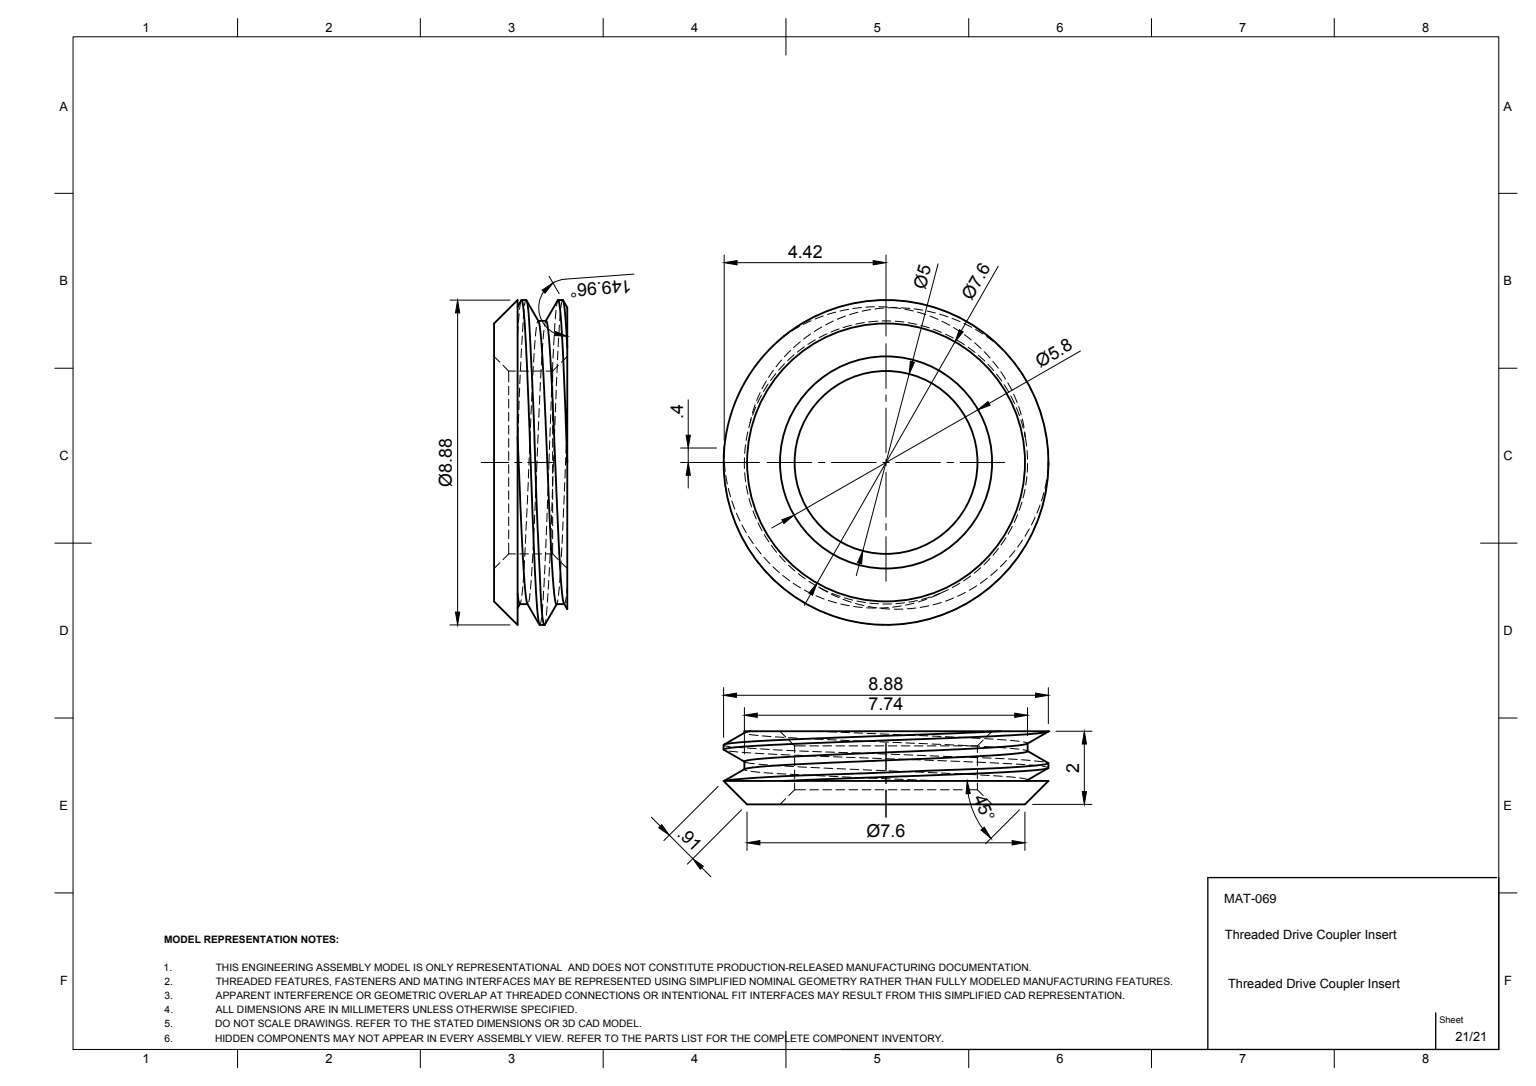
ISO-10303-21;
HEADER;
/* Generated by software containing ST-Developer
 * from STEP Tools, Inc. (www.steptools.com) 
 */

FILE_DESCRIPTION(
/* description */ ('CAx-IF Rec.Pracs.---Representation and Presentation of Product Manufa
cturing Information (PMI)---4.0---2014-10-13'),
/* implementation_level */ '2;1');

FILE_NAME(
/* name */ 'Threaded Drive Coupler Insert.step',
/* time_stamp */ '2026-10-24T15:08:39-07:00',
/* author */ (''),
/* organization */ (''),
/* preprocessor_version */ 'ST-DEVELOPER v20.2',
/* originating_system */ 'Autodesk Translation Framework v15.17.0.0',
/* authorisation */ '');

FILE_SCHEMA (('AP242_MANAGED_MODEL_BASED_3D_ENGINEERING_MIM_LF { 1 0 10303 442 2 1 4 }'));
ENDSEC;

DATA;
#10=MECHANICAL_DESIGN_GEOMETRIC_PRESENTATION_REPRESENTATION('',(#839),#50081);
#139=B_SPLINE_SURFACE_WITH_KNOTS('',3,3,((#49898,#49899,#49900,#49901,#49902,
#49903,#49904,#49905,#49906,#49907,#49908,#49909,#49910,#49911),(#49912,
#49913,#49914,#49915,#49916,#49917,#49918,#49919,#49920,#49921,#49922,#49923,
#49924,#49925),(#49926,#49927,#49928,#49929,#49930,#49931,#49932,#49933,
#49934,#49935,#49936,#49937,#49938,#49939),(#49940,#49941,#49942,#49943,
#49944,#49945,#49946,#49947,#49948,#49949,#49950,#49951,#49952,#49953)),
 .UNSPECIFIED.,.F.,.F.,.F.,(4,4),(4,1,1,1,1,1,1,1,1,1,1,4),(-0.000475468026429485,
0.0667497669206857),(7.06827384690996,8.03224682715675,8.99591018373647,
9.95957354031619,10.9232368968959,11.8869002534756,12.8505636100553,13.8142269666351,
14.7778903232148,15.7415536797945,16.7052170363742,17.6690343848084),
 .UNSPECIFIED.);
#140=B_SPLINE_SURFACE_WITH_KNOTS('',3,3,((#49960,#49961,#49962,#49963,#49964,
#49965,#49966,#49967,#49968,#49969,#49970,#49971,#49972,#49973),(#49974,
#49975,#49976,#49977,#49978,#49979,#49980,#49981,#49982,#49983,#49984,#49985,
#49986,#49987),(#49988,#49989,#49990,#49991,#49992,#49993,#49994,#49995,
#49996,#49997,#49998,#49999,#50000,#50001),(#50002,#50003,#50004,#50005,
#50006,#50007,#50008,#50009,#50010,#50011,#50012,#50013,#50014,#50015)),
 .UNSPECIFIED.,.F.,.F.,.F.,(4,4),(4,1,1,1,1,1,1,1,1,1,1,4),(-0.000976054051980672,
0.0662815922873265),(10.4983829434381,11.4623026957119,12.4259660522916,
13.3896294088713,14.353292765451,15.3169561220308,16.2806194786105,17.2442828351902,
18.2079461917699,19.1716095483496,20.1352729049293,21.0993547069101),
 .UNSPECIFIED.);
#588=B_SPLINE_CURVE_WITH_KNOTS('',3,(#49306,#49307,#49308,#49309,#49310,
#49311,#49312,#49313,#49314,#49315,#49316,#49317,#49318,#49319,#49320,#49321,
#49322,#49323,#49324,#49325,#49326,#49327,#49328,#49329,#49330),
 .UNSPECIFIED.,.F.,.F.,(4,3,3,3,3,3,3,3,4),(0.,0.160731090032336,0.25,0.407767129262868,
0.5,0.657767129262875,0.75,0.910731090032353,1.),.UNSPECIFIED.);
#589=B_SPLINE_CURVE_WITH_KNOTS('',3,(#49333,#49334,#49335,#49336,#49337,
#49338,#49339),.UNSPECIFIED.,.F.,.F.,(4,1,1,1,4),(0.,0.25,0.5,0.75,0.999999761822425),
 .UNSPECIFIED.);
#590=B_SPLINE_CURVE_WITH_KNOTS('',3,(#49345,#49346,#49347,#49348,#49349,
#49350,#49351,#49352,#49353,#49354,#49355,#49356,#49357,#49358,#49359,#49360,
#49361,#49362,#49363,#49364,#49365,#49366,#49367,#49368,#49369,#49370,#49371,
#49372,#49373,#49374,#49375,#49376,#49377,#49378,#49379,#49380,#49381,#49382,
#49383,#49384),.UNSPECIFIED.,.F.,.F.,(4,3,3,3,3,3,3,3,3,3,3,3,3,4),(0.235508041128149,
0.25,0.331910603091831,0.375,0.456895223609452,0.5,0.581895223609489,0.625,
0.706910603091898,0.75,0.831608731491742,0.875,0.958140783942944,0.999999441342508),
 .UNSPECIFIED.);
#591=B_SPLINE_CURVE_WITH_KNOTS('',3,(#49386,#49387,#49388,#49389),
 .UNSPECIFIED.,.F.,.F.,(4,4),(0.,0.987035809516257),.UNSPECIFIED.);
#592=B_SPLINE_CURVE_WITH_KNOTS('',3,(#49392,#49393,#49394,#49395,#49396,
#49397,#49398,#49399,#49400,#49401,#49402,#49403,#49404,#49405,#49406,#49407,
#49408,#49409,#49410,#49411,#49412,#49413,#49414,#49415),.UNSPECIFIED.,
 .F.,.F.,(4,2,2,2,2,2,2,2,2,2,2,4),(0.,0.100888900202487,0.125,0.22459286542628,
0.25,0.349878675008739,0.375,0.474842812735284,0.5,0.599842812735286,0.625,
0.715961029345133),.UNSPECIFIED.);
#593=B_SPLINE_CURVE_WITH_KNOTS('',3,(#49418,#49419,#49420,#49421,#49422,
#49423,#49424,#49425,#49426,#49427,#49428,#49429,#49430,#49431,#49432,#49433),
 .UNSPECIFIED.,.F.,.F.,(4,3,3,3,3,4),(0.715961029345133,0.75,0.849592865426306,
0.875,0.975888900203264,1.),.UNSPECIFIED.);
#594=B_SPLINE_CURVE_WITH_KNOTS('',3,(#49435,#49436,#49437,#49438,#49439,
#49440,#49441,#49442,#49443,#49444,#49445,#49446,#49447,#49448,#49449,#49450,
#49451,#49452,#49453,#49454,#49455,#49456,#49457,#49458,#49459),
 .UNSPECIFIED.,.F.,.F.,(4,3,3,3,3,3,3,3,4),(1.51276851349366E-6,0.156898311431348,
0.25,0.403657035544793,0.5,0.653657035544841,0.75,0.906896809192571,1.),
 .UNSPECIFIED.);
#595=B_SPLINE_CURVE_WITH_KNOTS('',3,(#49463,#49464,#49465,#49466,#49467,
#49468,#49469,#49470,#49471,#49472,#49473,#49474,#49475,#49476,#49477,#49478,
#49479,#49480,#49481),.UNSPECIFIED.,.F.,.F.,(4,3,3,3,3,3,4),(0.,0.25,0.491380882785342,
0.5,0.75,0.982966826876961,1.),.UNSPECIFIED.);
#596=B_SPLINE_CURVE_WITH_KNOTS('',3,(#49482,#49483,#49484,#49485,#49486,
#49487,#49488,#49489,#49490,#49491),.UNSPECIFIED.,.F.,.F.,(4,2,2,2,4),(0.,
0.0831407875458867,0.125,0.206497666001318,0.235508041094431),
 .UNSPECIFIED.);
#597=B_SPLINE_CURVE_WITH_KNOTS('',3,(#49494,#49495,#49496,#49497,#49498,
#49499,#49500,#49501,#49502,#49503,#49504,#49505,#49506,#49507,#49508,#49509,
#49510,#49511,#49512,#49513,#49514,#49515,#49516,#49517,#49518,#49519,#49520,
#49521,#49522,#49523,#49524,#49525,#49526,#49527,#49528,#49529,#49530,#49531,
#49532,#49533,#49534,#49535,#49536,#49537,#49538,#49539,#49540,#49541,#49542,
#49543,#49544,#49545,#49546,#49547,#49548,#49549,#49550,#49551,#49552,#49553,
#49554,#49555,#49556,#49557,#49558,#49559,#49560,#49561,#49562,#49563,#49564,
#49565,#49566,#49567,#49568,#49569,#49570,#49571,#49572,#49573,#49574,#49575,
#49576,#49577,#49578,#49579,#49580,#49581,#49582,#49583,#49584,#49585,#49586,
#49587,#49588,#49589),.UNSPECIFIED.,.F.,.F.,(4,2,2,2,2,2,2,2,2,2,2,2,2,
2,2,2,2,2,2,2,2,2,2,2,2,2,2,2,2,2,2,2,2,2,2,2,2,2,2,2,2,2,2,2,2,2,2,4),
(0.000203483817492821,0.0274848173325521,0.0563713830966491,0.167677917602274,
0.208184918082086,0.239301283250976,0.272826962459817,0.365270654699785,
0.43178988571008,0.47678039384355,0.587559073236576,0.632135152418474,0.664943612441571,
0.694797097900161,0.799548600392106,0.862971031190955,0.907614126172384,
0.988296557870209,1.06800029357004,1.09774395705088,1.13107244772413,1.22338481693792,
1.27276714107893,1.31911661255326,1.37385993664007,1.44604280082289,1.50302473070022,
1.53055325884595,1.56982870717352,1.63222593298961,1.71178156213431,1.75641486537916,
1.81980681943984,1.92449539617685,1.95434391906131,1.98714005868704,2.03169939876711,
2.14252612578957,2.18750485709249,2.25402546067906,2.3464077625176,2.37990009772018,
2.41102584148667,2.45156693199543,2.56907534347477,2.61465490234983,2.68897499185438,
2.74712781989908),.UNSPECIFIED.);
#598=B_SPLINE_CURVE_WITH_KNOTS('',3,(#49592,#49593,#49594,#49595,#49596,
#49597,#49598,#49599,#49600,#49601,#49602),.UNSPECIFIED.,.F.,.F.,(4,1,1,
1,1,1,1,1,4),(0.,0.125,0.25,0.375,0.5,0.625,0.75,0.875,0.999999067031556),
 .UNSPECIFIED.);
#599=B_SPLINE_CURVE_WITH_KNOTS('',3,(#49615,#49616,#49617,#49618,#49619,
#49620,#49621,#49622,#49623,#49624,#49625,#49626,#49627,#49628,#49629,#49630,
#49631,#49632,#49633,#49634,#49635,#49636,#49637,#49638,#49639,#49640,#49641,
#49642,#49643,#49644,#49645,#49646,#49647,#49648,#49649,#49650,#49651,#49652,
#49653,#49654,#49655,#49656,#49657,#49658,#49659,#49660,#49661,#49662,#49663,
#49664,#49665,#49666,#49667,#49668,#49669,#49670,#49671,#49672,#49673,#49674,
#49675,#49676,#49677,#49678,#49679,#49680,#49681,#49682,#49683,#49684,#49685,
#49686,#49687,#49688,#49689,#49690,#49691,#49692,#49693,#49694,#49695,#49696,
#49697,#49698,#49699,#49700,#49701,#49702,#49703,#49704,#49705),
 .UNSPECIFIED.,.F.,.F.,(4,3,3,3,3,3,3,3,3,3,3,3,3,3,3,3,3,3,3,3,3,3,3,3,
3,3,3,3,3,3,4),(0.,0.0549095480248197,0.0909168947914259,0.127664846372719,
0.147588217015191,0.152802982426264,0.157890055006788,0.195093310789768,
0.232935081254819,0.292943797457197,0.305066964469618,0.310416184503556,
0.349172960287603,0.387949178487593,0.446438776652271,0.460993647480443,
0.469743525078789,0.474867539044195,0.512454117005302,0.550939413816203,
0.624355350952517,0.633225532922949,0.64024307789027,0.680180338798595,
0.720316379107474,0.73809145220851,0.748199996374111,0.754956026360989,
0.795541316014259,0.835496820076563,0.862516963915765),.UNSPECIFIED.);
#600=B_SPLINE_CURVE_WITH_KNOTS('',3,(#49706,#49707,#49708,#49709,#49710,
#49711,#49712,#49713,#49714,#49715,#49716,#49717,#49718,#49719,#49720,#49721,
#49722,#49723,#49724,#49725,#49726,#49727,#49728,#49729,#49730,#49731,#49732,
#49733,#49734,#49735,#49736,#49737,#49738,#49739,#49740,#49741,#49742,#49743,
#49744,#49745,#49746,#49747,#49748,#49749,#49750,#49751,#49752,#49753,#49754,
#49755,#49756,#49757,#49758,#49759,#49760,#49761,#49762,#49763,#49764,#49765,
#49766,#49767,#49768,#49769,#49770,#49771,#49772),.UNSPECIFIED.,.F.,.F.,
(4,3,3,3,3,3,3,3,3,3,3,3,3,3,3,3,3,3,3,3,3,3,4),(0.,0.0399225644477167,
0.0623885722514162,0.164012510354697,0.170043304514999,0.174785078605868,
0.294020040644772,0.316832921701425,0.3295965682445,0.337876395007978,0.382194010439746,
0.420601788797671,0.476523089097994,0.50063461453704,0.506312621506711,
0.652610410209141,0.659762241707176,0.665735072710524,0.763244547674934,
0.769629684943624,0.806337248425914,0.842085556810208,0.865008878888598),
 .UNSPECIFIED.);
#601=B_SPLINE_CURVE_WITH_KNOTS('',3,(#49773,#49774,#49775,#49776,#49777,
#49778),.UNSPECIFIED.,.F.,.F.,(4,2,4),(3.98711970495987E-6,0.000952908437083531,
0.00170790873623591),.UNSPECIFIED.);
#602=B_SPLINE_CURVE_WITH_KNOTS('',3,(#49790,#49791,#49792,#49793,#49794,
#49795,#49796,#49797,#49798,#49799,#49800,#49801,#49802,#49803,#49804,#49805,
#49806,#49807,#49808,#49809,#49810,#49811,#49812,#49813,#49814,#49815,#49816,
#49817,#49818,#49819,#49820,#49821,#49822,#49823,#49824,#49825,#49826,#49827,
#49828,#49829,#49830,#49831,#49832,#49833,#49834,#49835,#49836,#49837,#49838,
#49839,#49840,#49841,#49842,#49843,#49844),.UNSPECIFIED.,.F.,.F.,(4,3,3,
3,3,3,3,3,3,3,3,3,3,3,3,3,3,3,4),(-0.854915111010944,-0.822925495947057,
-0.800365095426597,-0.75633398547855,-0.748469100844136,-0.742037773638304,
-0.645772245378637,-0.632162604915744,-0.459766793866444,-0.38991304085735,
-0.38779448365469,-0.315984565381592,-0.310449867153767,-0.30493629935315,
-0.167082233063672,-0.154397747235191,-0.14936263256871,-0.00258798757819179,
0.),.UNSPECIFIED.);
#603=B_SPLINE_CURVE_WITH_KNOTS('',3,(#49845,#49846,#49847,#49848,#49849,
#49850,#49851,#49852,#49853,#49854,#49855,#49856,#49857,#49858,#49859,#49860,
#49861,#49862,#49863,#49864,#49865,#49866,#49867,#49868,#49869,#49870,#49871,
#49872,#49873,#49874,#49875,#49876,#49877,#49878,#49879,#49880,#49881,#49882,
#49883,#49884,#49885,#49886,#49887,#49888,#49889,#49890,#49891,#49892,#49893,
#49894,#49895,#49896),.UNSPECIFIED.,.F.,.F.,(4,3,3,3,3,3,3,3,3,3,3,3,3,
3,3,3,3,4),(-0.865008878888613,-0.810020253230451,-0.667799397338663,-0.661220440996107,
-0.656149039337886,-0.510599083577838,-0.503912127317129,-0.497491726604393,
-0.417709321956839,-0.355786573118897,-0.34402092652179,-0.338375890722606,
-0.294627424667398,-0.255060288195652,-0.188293674813484,-0.175394629447954,
-0.00556396810409777,0.),.UNSPECIFIED.);
#604=B_SPLINE_CURVE_WITH_KNOTS('',3,(#49954,#49955,#49956,#49957,#49958,
#49959),.UNSPECIFIED.,.F.,.F.,(4,2,4),(0.000198558815412191,0.00408016890061404,
0.00800258217218409),.UNSPECIFIED.);
#662=CONICAL_SURFACE('',#11001,0.0027,0.785398163397448);
#663=CONICAL_SURFACE('',#11007,0.0027,0.785398163397448);
#664=CONICAL_SURFACE('',#11014,0.0039,0.785398163397448);
#767=FACE_BOUND('',#2235,.T.);
#768=FACE_BOUND('',#2238,.T.);
#799=SHAPE_REPRESENTATION_RELATIONSHIP('SRR','None',#50167,#819);
#819=ADVANCED_BREP_SHAPE_REPRESENTATION('',(#859),#50080);
#839=STYLED_ITEM('',(#50261),#859);
#859=MANIFOLD_SOLID_BREP('Body1',#9884);
#1099=PLANE('',#11006);
#1100=PLANE('',#11009);
#1101=PLANE('',#11011);
#1630=FACE_OUTER_BOUND('',#2228,.T.);
#1631=FACE_OUTER_BOUND('',#2229,.T.);
#1632=FACE_OUTER_BOUND('',#2230,.T.);
#1633=FACE_OUTER_BOUND('',#2231,.T.);
#1634=FACE_OUTER_BOUND('',#2232,.T.);
#1635=FACE_OUTER_BOUND('',#2233,.T.);
#1636=FACE_OUTER_BOUND('',#2234,.T.);
#1637=FACE_OUTER_BOUND('',#2236,.T.);
#1638=FACE_OUTER_BOUND('',#2237,.T.);
#1639=FACE_OUTER_BOUND('',#2239,.T.);
#1640=FACE_OUTER_BOUND('',#2240,.T.);
#1641=FACE_OUTER_BOUND('',#2241,.T.);
#1642=FACE_OUTER_BOUND('',#2242,.T.);
#2228=EDGE_LOOP('',(#9078,#9079,#9080,#9081));
#2229=EDGE_LOOP('',(#9082,#9083,#9084,#9085,#9086));
#2230=EDGE_LOOP('',(#9087,#9088,#9089,#9090,#9091,#9092));
#2231=EDGE_LOOP('',(#9093,#9094,#9095,#9096));
#2232=EDGE_LOOP('',(#9097,#9098,#9099,#9100));
#2233=EDGE_LOOP('',(#9101,#9102,#9103,#9104));
#2234=EDGE_LOOP('',(#9105,#9106,#9107,#9108,#9109));
#2235=EDGE_LOOP('',(#9110));
#2236=EDGE_LOOP('',(#9111,#9112,#9113,#9114));
#2237=EDGE_LOOP('',(#9115));
#2238=EDGE_LOOP('',(#9116));
#2239=EDGE_LOOP('',(#9117,#9118,#9119,#9120,#9121));
#2240=EDGE_LOOP('',(#9122,#9123,#9124,#9125,#9126,#9127,#9128,#9129,#9130,
#9131));
#2241=EDGE_LOOP('',(#9132,#9133,#9134,#9135,#9136,#9137,#9138));
#2242=EDGE_LOOP('',(#9139,#9140,#9141,#9142,#9143,#9144,#9145));
#2815=LINE('',#49304,#3393);
#2816=LINE('',#49343,#3394);
#2817=LINE('',#49607,#3395);
#2818=LINE('',#49611,#3396);
#2819=LINE('',#49781,#3397);
#2820=LINE('',#50017,#3398);
#3393=VECTOR('',#13383,0.004442);
#3394=VECTOR('',#13388,0.003872);
#3395=VECTOR('',#13403,0.0027);
#3396=VECTOR('',#13408,0.0025);
#3397=VECTOR('',#13415,0.0027);
#3398=VECTOR('',#13430,0.0039);
#3761=CIRCLE('',#10994,0.00444200000001);
#3762=CIRCLE('',#10996,0.00387200000001);
#3763=CIRCLE('',#10998,0.00387200000001);
#3764=CIRCLE('',#11000,0.00444200000001);
#3765=CIRCLE('',#11002,0.00250000000001);
#3766=CIRCLE('',#11003,0.00290000000001);
#3767=CIRCLE('',#11005,0.00250000000001);
#3768=CIRCLE('',#11008,0.00290000000001);
#3769=CIRCLE('',#11010,0.00380000000001);
#3770=CIRCLE('',#11012,0.00444200000001);
#3771=CIRCLE('',#11013,0.00444200000001);
#4743=VERTEX_POINT('',#49302);
#4744=VERTEX_POINT('',#49303);
#4745=VERTEX_POINT('',#49305);
#4746=VERTEX_POINT('',#49331);
#4747=VERTEX_POINT('',#49341);
#4748=VERTEX_POINT('',#49342);
#4749=VERTEX_POINT('',#49344);
#4750=VERTEX_POINT('',#49385);
#4751=VERTEX_POINT('',#49390);
#4752=VERTEX_POINT('',#49417);
#4753=VERTEX_POINT('',#49434);
#4754=VERTEX_POINT('',#49460);
#4755=VERTEX_POINT('',#49462);
#4756=VERTEX_POINT('',#49493);
#4757=VERTEX_POINT('',#49590);
#4758=VERTEX_POINT('',#49604);
#4759=VERTEX_POINT('',#49606);
#4760=VERTEX_POINT('',#49610);
#4761=VERTEX_POINT('',#49614);
#4762=VERTEX_POINT('',#49780);
#4763=VERTEX_POINT('',#49784);
#4764=VERTEX_POINT('',#49787);
#4765=VERTEX_POINT('',#49788);
#6192=EDGE_CURVE('',#4743,#4744,#2815,.T.);
#6193=EDGE_CURVE('',#4743,#4745,#588,.T.);
#6194=EDGE_CURVE('',#4745,#4746,#3761,.T.);
#6195=EDGE_CURVE('',#4746,#4744,#589,.T.);
#6196=EDGE_CURVE('',#4747,#4748,#2816,.T.);
#6197=EDGE_CURVE('',#4749,#4747,#590,.F.);
#6198=EDGE_CURVE('',#4750,#4749,#591,.F.);
#6199=EDGE_CURVE('',#4751,#4750,#3762,.T.);
#6200=EDGE_CURVE('',#4751,#4748,#592,.T.);
#6201=EDGE_CURVE('',#4748,#4752,#593,.T.);
#6202=EDGE_CURVE('',#4752,#4753,#594,.T.);
#6203=EDGE_CURVE('',#4754,#4753,#3763,.T.);
#6204=EDGE_CURVE('',#4755,#4754,#595,.F.);
#6205=EDGE_CURVE('',#4747,#4755,#596,.F.);
#6206=EDGE_CURVE('',#4744,#4756,#597,.T.);
#6207=EDGE_CURVE('',#4757,#4756,#3764,.T.);
#6208=EDGE_CURVE('',#4757,#4743,#598,.T.);
#6209=EDGE_CURVE('',#4758,#4758,#3765,.T.);
#6210=EDGE_CURVE('',#4758,#4759,#2817,.T.);
#6211=EDGE_CURVE('',#4759,#4759,#3766,.T.);
#6212=EDGE_CURVE('',#4758,#4760,#2818,.T.);
#6213=EDGE_CURVE('',#4760,#4760,#3767,.T.);
#6214=EDGE_CURVE('',#4761,#4746,#599,.T.);
#6215=EDGE_CURVE('',#4745,#4751,#600,.T.);
#6216=EDGE_CURVE('',#4761,#4750,#601,.T.);
#6217=EDGE_CURVE('',#4760,#4762,#2819,.T.);
#6218=EDGE_CURVE('',#4762,#4762,#3768,.T.);
#6219=EDGE_CURVE('',#4763,#4763,#3769,.T.);
#6220=EDGE_CURVE('',#4764,#4765,#3770,.T.);
#6221=EDGE_CURVE('',#4764,#4754,#602,.T.);
#6222=EDGE_CURVE('',#4753,#4757,#603,.T.);
#6223=EDGE_CURVE('',#4765,#4757,#3771,.T.);
#6224=EDGE_CURVE('',#4756,#4764,#604,.T.);
#6225=EDGE_CURVE('',#4765,#4763,#2820,.T.);
#9078=ORIENTED_EDGE('',*,*,#6192,.F.);
#9079=ORIENTED_EDGE('',*,*,#6193,.T.);
#9080=ORIENTED_EDGE('',*,*,#6194,.T.);
#9081=ORIENTED_EDGE('',*,*,#6195,.T.);
#9082=ORIENTED_EDGE('',*,*,#6196,.F.);
#9083=ORIENTED_EDGE('',*,*,#6197,.F.);
#9084=ORIENTED_EDGE('',*,*,#6198,.F.);
#9085=ORIENTED_EDGE('',*,*,#6199,.F.);
#9086=ORIENTED_EDGE('',*,*,#6200,.T.);
#9087=ORIENTED_EDGE('',*,*,#6196,.T.);
#9088=ORIENTED_EDGE('',*,*,#6201,.T.);
#9089=ORIENTED_EDGE('',*,*,#6202,.T.);
#9090=ORIENTED_EDGE('',*,*,#6203,.F.);
#9091=ORIENTED_EDGE('',*,*,#6204,.F.);
#9092=ORIENTED_EDGE('',*,*,#6205,.F.);
#9093=ORIENTED_EDGE('',*,*,#6192,.T.);
#9094=ORIENTED_EDGE('',*,*,#6206,.T.);
#9095=ORIENTED_EDGE('',*,*,#6207,.F.);
#9096=ORIENTED_EDGE('',*,*,#6208,.T.);
#9097=ORIENTED_EDGE('',*,*,#6209,.T.);
#9098=ORIENTED_EDGE('',*,*,#6210,.T.);
#9099=ORIENTED_EDGE('',*,*,#6211,.T.);
#9100=ORIENTED_EDGE('',*,*,#6210,.F.);
#9101=ORIENTED_EDGE('',*,*,#6209,.F.);
#9102=ORIENTED_EDGE('',*,*,#6212,.T.);
#9103=ORIENTED_EDGE('',*,*,#6213,.F.);
#9104=ORIENTED_EDGE('',*,*,#6212,.F.);
#9105=ORIENTED_EDGE('',*,*,#6214,.T.);
#9106=ORIENTED_EDGE('',*,*,#6194,.F.);
#9107=ORIENTED_EDGE('',*,*,#6215,.T.);
#9108=ORIENTED_EDGE('',*,*,#6199,.T.);
#9109=ORIENTED_EDGE('',*,*,#6216,.F.);
#9110=ORIENTED_EDGE('',*,*,#6211,.F.);
#9111=ORIENTED_EDGE('',*,*,#6213,.T.);
#9112=ORIENTED_EDGE('',*,*,#6217,.T.);
#9113=ORIENTED_EDGE('',*,*,#6218,.T.);
#9114=ORIENTED_EDGE('',*,*,#6217,.F.);
#9115=ORIENTED_EDGE('',*,*,#6219,.F.);
#9116=ORIENTED_EDGE('',*,*,#6218,.F.);
#9117=ORIENTED_EDGE('',*,*,#6220,.F.);
#9118=ORIENTED_EDGE('',*,*,#6221,.T.);
#9119=ORIENTED_EDGE('',*,*,#6203,.T.);
#9120=ORIENTED_EDGE('',*,*,#6222,.T.);
#9121=ORIENTED_EDGE('',*,*,#6223,.F.);
#9122=ORIENTED_EDGE('',*,*,#6221,.F.);
#9123=ORIENTED_EDGE('',*,*,#6224,.F.);
#9124=ORIENTED_EDGE('',*,*,#6206,.F.);
#9125=ORIENTED_EDGE('',*,*,#6195,.F.);
#9126=ORIENTED_EDGE('',*,*,#6214,.F.);
#9127=ORIENTED_EDGE('',*,*,#6216,.T.);
#9128=ORIENTED_EDGE('',*,*,#6198,.T.);
#9129=ORIENTED_EDGE('',*,*,#6197,.T.);
#9130=ORIENTED_EDGE('',*,*,#6205,.T.);
#9131=ORIENTED_EDGE('',*,*,#6204,.T.);
#9132=ORIENTED_EDGE('',*,*,#6222,.F.);
#9133=ORIENTED_EDGE('',*,*,#6202,.F.);
#9134=ORIENTED_EDGE('',*,*,#6201,.F.);
#9135=ORIENTED_EDGE('',*,*,#6200,.F.);
#9136=ORIENTED_EDGE('',*,*,#6215,.F.);
#9137=ORIENTED_EDGE('',*,*,#6193,.F.);
#9138=ORIENTED_EDGE('',*,*,#6208,.F.);
#9139=ORIENTED_EDGE('',*,*,#6220,.T.);
#9140=ORIENTED_EDGE('',*,*,#6225,.T.);
#9141=ORIENTED_EDGE('',*,*,#6219,.T.);
#9142=ORIENTED_EDGE('',*,*,#6225,.F.);
#9143=ORIENTED_EDGE('',*,*,#6223,.T.);
#9144=ORIENTED_EDGE('',*,*,#6207,.T.);
#9145=ORIENTED_EDGE('',*,*,#6224,.T.);
#9319=CYLINDRICAL_SURFACE('',#10993,0.004442);
#9320=CYLINDRICAL_SURFACE('',#10995,0.003872);
#9321=CYLINDRICAL_SURFACE('',#10997,0.003872);
#9322=CYLINDRICAL_SURFACE('',#10999,0.004442);
#9323=CYLINDRICAL_SURFACE('',#11004,0.0025);
#9852=ADVANCED_FACE('',(#1630),#9319,.T.);
#9853=ADVANCED_FACE('',(#1631),#9320,.T.);
#9854=ADVANCED_FACE('',(#1632),#9321,.T.);
#9855=ADVANCED_FACE('',(#1633),#9322,.T.);
#9856=ADVANCED_FACE('',(#1634),#662,.F.);
#9857=ADVANCED_FACE('',(#1635),#9323,.F.);
#9858=ADVANCED_FACE('',(#1636,#767),#1099,.F.);
#9859=ADVANCED_FACE('',(#1637),#663,.F.);
#9860=ADVANCED_FACE('',(#1638,#768),#1100,.T.);
#9861=ADVANCED_FACE('',(#1639),#1101,.F.);
#9862=ADVANCED_FACE('',(#1640),#139,.F.);
#9863=ADVANCED_FACE('',(#1641),#140,.F.);
#9864=ADVANCED_FACE('',(#1642),#664,.T.);
#9884=CLOSED_SHELL('',(#9852,#9853,#9854,#9855,#9856,#9857,#9858,#9859,
#9860,#9861,#9862,#9863,#9864));
#10992=AXIS2_PLACEMENT_3D('',#49300,#13379,#13380);
#10993=AXIS2_PLACEMENT_3D('',#49301,#13381,#13382);
#10994=AXIS2_PLACEMENT_3D('',#49332,#13384,#13385);
#10995=AXIS2_PLACEMENT_3D('',#49340,#13386,#13387);
#10996=AXIS2_PLACEMENT_3D('',#49391,#13389,#13390);
#10997=AXIS2_PLACEMENT_3D('',#49416,#13391,#13392);
#10998=AXIS2_PLACEMENT_3D('',#49461,#13393,#13394);
#10999=AXIS2_PLACEMENT_3D('',#49492,#13395,#13396);
#11000=AXIS2_PLACEMENT_3D('',#49591,#13397,#13398);
#11001=AXIS2_PLACEMENT_3D('',#49603,#13399,#13400);
#11002=AXIS2_PLACEMENT_3D('',#49605,#13401,#13402);
#11003=AXIS2_PLACEMENT_3D('',#49608,#13404,#13405);
#11004=AXIS2_PLACEMENT_3D('',#49609,#13406,#13407);
#11005=AXIS2_PLACEMENT_3D('',#49612,#13409,#13410);
#11006=AXIS2_PLACEMENT_3D('',#49613,#13411,#13412);
#11007=AXIS2_PLACEMENT_3D('',#49779,#13413,#13414);
#11008=AXIS2_PLACEMENT_3D('',#49782,#13416,#13417);
#11009=AXIS2_PLACEMENT_3D('',#49783,#13418,#13419);
#11010=AXIS2_PLACEMENT_3D('',#49785,#13420,#13421);
#11011=AXIS2_PLACEMENT_3D('',#49786,#13422,#13423);
#11012=AXIS2_PLACEMENT_3D('',#49789,#13424,#13425);
#11013=AXIS2_PLACEMENT_3D('',#49897,#13426,#13427);
#11014=AXIS2_PLACEMENT_3D('',#50016,#13428,#13429);
#13379=DIRECTION('axis',(0.,0.,1.));
#13380=DIRECTION('refdir',(1.,0.,0.));
#13381=DIRECTION('center_axis',(0.,1.,1.09634523681734E-15));
#13382=DIRECTION('ref_axis',(1.,0.,0.));
#13383=DIRECTION('',(0.,-1.,-1.09634523681734E-15));
#13384=DIRECTION('center_axis',(0.,1.,1.09634523681734E-15));
#13385=DIRECTION('ref_axis',(1.,0.,0.));
#13386=DIRECTION('center_axis',(0.,1.,1.09634523681734E-15));
#13387=DIRECTION('ref_axis',(0.0907903645015774,-1.09181736006036E-15,0.995870026516347));
#13388=DIRECTION('',(0.,-1.,-1.09634523681734E-15));
#13389=DIRECTION('center_axis',(0.,-1.,-1.09634523681734E-15));
#13390=DIRECTION('ref_axis',(1.,2.83177819361768E-27,-2.58292561368557E-12));
#13391=DIRECTION('center_axis',(0.,1.,1.09634523681734E-15));
#13392=DIRECTION('ref_axis',(0.0907903645015774,-1.09181736006036E-15,0.995870026516347));
#13393=DIRECTION('center_axis',(0.,1.,1.09634523681734E-15));
#13394=DIRECTION('ref_axis',(1.,2.83177819361768E-27,-2.58292561368557E-12));
#13395=DIRECTION('center_axis',(0.,1.,1.09634523681734E-15));
#13396=DIRECTION('ref_axis',(1.,0.,0.));
#13397=DIRECTION('center_axis',(0.,1.,1.09634523681734E-15));
#13398=DIRECTION('ref_axis',(1.,0.,0.));
#13399=DIRECTION('center_axis',(0.,-1.,-1.09634523681734E-15));
#13400=DIRECTION('ref_axis',(1.,0.,0.));
#13401=DIRECTION('center_axis',(0.,1.,1.09634523681734E-15));
#13402=DIRECTION('ref_axis',(1.,0.,0.));
#13403=DIRECTION('',(-0.707106781186547,-0.707106781186548,-8.61828757098662E-16));
#13404=DIRECTION('center_axis',(0.,-1.,-1.09634523681734E-15));
#13405=DIRECTION('ref_axis',(1.,0.,0.));
#13406=DIRECTION('center_axis',(0.,1.,1.09634523681734E-15));
#13407=DIRECTION('ref_axis',(1.,0.,0.));
#13408=DIRECTION('',(0.,1.,1.09634523681734E-15));
#13409=DIRECTION('center_axis',(0.,-1.,-1.09634523681734E-15));
#13410=DIRECTION('ref_axis',(1.,0.,0.));
#13411=DIRECTION('center_axis',(0.,1.,1.09634523681734E-15));
#13412=DIRECTION('ref_axis',(1.,0.,0.));
#13413=DIRECTION('center_axis',(0.,1.,1.09634523681734E-15));
#13414=DIRECTION('ref_axis',(1.,0.,0.));
#13415=DIRECTION('',(-0.707106781186547,0.707106781186548,8.61828757098662E-16));
#13416=DIRECTION('center_axis',(0.,1.,1.09634523681734E-15));
#13417=DIRECTION('ref_axis',(1.,0.,0.));
#13418=DIRECTION('center_axis',(0.,1.,1.09634523681734E-15));
#13419=DIRECTION('ref_axis',(1.,0.,0.));
#13420=DIRECTION('center_axis',(0.,-1.,-1.09634523681734E-15));
#13421=DIRECTION('ref_axis',(1.,0.,0.));
#13422=DIRECTION('center_axis',(0.,1.,1.09634523681734E-15));
#13423=DIRECTION('ref_axis',(1.,0.,0.));
#13424=DIRECTION('center_axis',(0.,1.,1.09634523681734E-15));
#13425=DIRECTION('ref_axis',(1.,0.,0.));
#13426=DIRECTION('center_axis',(0.,1.,1.09634523681734E-15));
#13427=DIRECTION('ref_axis',(1.,0.,0.));
#13428=DIRECTION('center_axis',(0.,-1.,-1.09634523681734E-15));
#13429=DIRECTION('ref_axis',(1.,0.,0.));
#13430=DIRECTION('',(0.707106781186547,0.707106781186548,8.61828757098662E-16));
#49300=CARTESIAN_POINT('',(0.,0.,0.));
#49301=CARTESIAN_POINT('Origin',(0.,0.0135212256101277,-0.0121758532865581));
#49302=CARTESIAN_POINT('',(-0.00444207914276344,0.0140214195594295,-0.0121760606789385));
#49303=CARTESIAN_POINT('',(-0.00444199985070438,0.0138962255208211,-0.0121770049558098));
#49304=CARTESIAN_POINT('',(-0.004442,0.0135212256101277,-0.0121758532865581));
#49305=CARTESIAN_POINT('',(0.00444199999990267,0.0135213203764857,-0.0121758826923265));
#49306=CARTESIAN_POINT('Ctrl Pts',(-0.00444199963579549,0.0140212256101377,
-0.01217765206189));
#49307=CARTESIAN_POINT('Ctrl Pts',(-0.00444169691062519,0.0139944421724318,
-0.0129252190717282));
#49308=CARTESIAN_POINT('Ctrl Pts',(-0.00424834946874033,0.0139676587347259,
-0.0136731455972233));
#49309=CARTESIAN_POINT('Ctrl Pts',(-0.00388623378020746,0.0139408752970199,
-0.0143272600369367));
#49310=CARTESIAN_POINT('Ctrl Pts',(-0.0036851172893592,0.0139259999652549,
-0.0146905505678201));
#49311=CARTESIAN_POINT('Ctrl Pts',(-0.00343290851149104,0.0139111246334898,
-0.0150250580165878));
#49312=CARTESIAN_POINT('Ctrl Pts',(-0.00314001943231033,0.0138962493017247,
-0.0153177702117351));
#49313=CARTESIAN_POINT('Ctrl Pts',(-0.00262238939480316,0.0138699597638524,
-0.0158350876377611));
#49314=CARTESIAN_POINT('Ctrl Pts',(-0.00197179931976566,0.0138436702259802,
-0.016223435502831));
#49315=CARTESIAN_POINT('Ctrl Pts',(-0.00126781229392693,0.0138173806881079,
-0.0164330843100483));
#49316=CARTESIAN_POINT('Ctrl Pts',(-0.000856251630700209,0.0138020114565092,
-0.0165556479354792));
#49317=CARTESIAN_POINT('Ctrl Pts',(-0.000427119037945985,0.0137866422249104,
-0.0166179384412321));
#49318=CARTESIAN_POINT('Ctrl Pts',(8.84684800475695E-7,0.0137712729933117,
-0.0166178531984596));
#49319=CARTESIAN_POINT('Ctrl Pts',(0.000732998063814579,0.0137449834554394,
-0.0166177073881058));
#49320=CARTESIAN_POINT('Ctrl Pts',(0.00146774307875059,0.0137186939175672,
-0.0164322051299338));
#49321=CARTESIAN_POINT('Ctrl Pts',(0.00211372343292607,0.0136924043796949,
-0.0160827110071693));
#49322=CARTESIAN_POINT('Ctrl Pts',(0.0024913725844557,0.0136770351480962,
-0.0158783918540039));
#49323=CARTESIAN_POINT('Ctrl Pts',(0.00283877742384937,0.0136616659164974,
-0.0156190707264348));
#49324=CARTESIAN_POINT('Ctrl Pts',(0.00314127069427827,0.0136462966848987,
-0.0153165192072298));
#49325=CARTESIAN_POINT('Ctrl Pts',(0.00366841543882451,0.0136195132471928,
-0.0147892729545205));
#49326=CARTESIAN_POINT('Ctrl Pts',(0.00406108394339532,0.0135927298094869,
-0.0141249068751873));
#49327=CARTESIAN_POINT('Ctrl Pts',(0.00426828489609652,0.0135659463717809,
-0.0134059378550957));
#49328=CARTESIAN_POINT('Ctrl Pts',(0.00438336283893988,0.0135510710400159,
-0.0130066275492229));
#49329=CARTESIAN_POINT('Ctrl Pts',(0.00444199725134734,0.0135361957082508,
-0.0125910761533599));
#49330=CARTESIAN_POINT('Ctrl Pts',(0.00444199999990267,0.0135213203764857,
-0.0121758826923265));
#49331=CARTESIAN_POINT('',(0.00314096832203065,0.0135212256101277,-0.0153168216085888));
#49332=CARTESIAN_POINT('Origin',(0.,0.0135212256101277,-0.0121758532865581));
#49333=CARTESIAN_POINT('Ctrl Pts',(0.00314096832203065,0.0135212256101277,
-0.0153168216085887));
#49334=CARTESIAN_POINT('Ctrl Pts',(0.00252430835006519,0.0135524756101285,
-0.0159334815805542));
#49335=CARTESIAN_POINT('Ctrl Pts',(0.000918657482604838,0.0136149756101302,
-0.0167914720831634));
#49336=CARTESIAN_POINT('Ctrl Pts',(-0.00180052581929913,0.0137087256101327,
-0.0165242980061952));
#49337=CARTESIAN_POINT('Ctrl Pts',(-0.00391264718618217,0.013802475580363,
-0.0147910125690047));
#49338=CARTESIAN_POINT('Ctrl Pts',(-0.00444177373170171,0.0138649755505925,
-0.0130490929893534));
#49339=CARTESIAN_POINT('Ctrl Pts',(-0.00444199985070438,0.0138962255208211,
-0.0121770049558098));
#49340=CARTESIAN_POINT('Origin',(0.,0.0118503152635658,-0.0121758532865581));
#49341=CARTESIAN_POINT('',(-0.000351540290533838,0.0143316213495927,-0.0160318620293038));
#49342=CARTESIAN_POINT('',(-0.000351540291350108,0.0141148214918298,-0.0160318620292294));
#49343=CARTESIAN_POINT('',(-0.000351540291350108,0.0118503152635658,-0.0160318620292294));
#49344=CARTESIAN_POINT('',(-0.00387240384587368,0.013567201943267,-0.0121762315324215));
#49345=CARTESIAN_POINT('Ctrl Pts',(-0.000351540290533835,0.0143316213495927,
-0.0160318620293038));
#49346=CARTESIAN_POINT('Ctrl Pts',(-0.000234595974335966,0.0143267909932129,
-0.0160425234778728));
#49347=CARTESIAN_POINT('Ctrl Pts',(-0.000117241700454775,0.0143219606368333,
-0.0160478536951273));
#49348=CARTESIAN_POINT('Ctrl Pts',(1.34925462922058E-8,0.0143171302804535,
-0.0160478532865346));
#49349=CARTESIAN_POINT('Ctrl Pts',(0.000662756442570941,0.0142898284223879,
-0.0160478509771105));
#49350=CARTESIAN_POINT('Ctrl Pts',(0.00132773602328349,0.0142625265643224,
-0.0158733453024538));
#49351=CARTESIAN_POINT('Ctrl Pts',(0.00190636873638902,0.0142352247062569,
-0.01554603759026));
#49352=CARTESIAN_POINT('Ctrl Pts',(0.00221076076499003,0.0142208624557775,
-0.0153738560729781));
#49353=CARTESIAN_POINT('Ctrl Pts',(0.002491395206892,0.0142065002052982,
-0.0151602947490979));
#49354=CARTESIAN_POINT('Ctrl Pts',(0.00273792720729818,0.0141921379548189,
-0.0149137609927338));
#49355=CARTESIAN_POINT('Ctrl Pts',(0.00320648315722661,0.0141648412229327,
-0.0144452017054515));
#49356=CARTESIAN_POINT('Ctrl Pts',(0.00355326033299318,0.0141375444910466,
-0.0138517103965861));
#49357=CARTESIAN_POINT('Ctrl Pts',(0.00373099531145518,0.0141102477591604,
-0.0132112556170072));
#49358=CARTESIAN_POINT('Ctrl Pts',(0.00382454443637019,0.0140958803825017,
-0.0128741583011288));
#49359=CARTESIAN_POINT('Ctrl Pts',(0.00387200126873256,0.014081513005843,
-0.0125245939908508));
#49360=CARTESIAN_POINT('Ctrl Pts',(0.00387199999997438,0.0140671456291843,
-0.0121758392003525));
#49361=CARTESIAN_POINT('Ctrl Pts',(0.0038719975894472,0.0140398488972981,
-0.0115132362606235));
#49362=CARTESIAN_POINT('Ctrl Pts',(0.00369756338123366,0.0140125521654119,
-0.0108483757539588));
#49363=CARTESIAN_POINT('Ctrl Pts',(0.00337037109597679,0.0139852554335258,
-0.0102698148096631));
#49364=CARTESIAN_POINT('Ctrl Pts',(0.00319815653118179,0.0139708880568671,
-0.00996529472860113));
#49365=CARTESIAN_POINT('Ctrl Pts',(0.00298452907348282,0.0139565206802084,
-0.00968454561436105));
#49366=CARTESIAN_POINT('Ctrl Pts',(0.00273790728639367,0.0139421533035497,
-0.00943792565948093));
#49367=CARTESIAN_POINT('Ctrl Pts',(0.00226925993434475,0.0139148514454841,
-0.00896928178911916));
#49368=CARTESIAN_POINT('Ctrl Pts',(0.00167564221543866,0.0138875495874186,
-0.00862246838979723));
#49369=CARTESIAN_POINT('Ctrl Pts',(0.00103505110354679,0.013860247729353,
-0.00844476052262867));
#49370=CARTESIAN_POINT('Ctrl Pts',(0.000698065614071849,0.0138458854788737,
-0.0083512765958466));
#49371=CARTESIAN_POINT('Ctrl Pts',(0.000348623871723006,0.0138315232283944,
-0.00830385196479697));
#49372=CARTESIAN_POINT('Ctrl Pts',(-1.46798648791328E-8,0.0138171609779151,
-0.00830385328658593));
#49373=CARTESIAN_POINT('Ctrl Pts',(-0.000660315171071245,0.0137899597375385,
-0.00830385578997487));
#49374=CARTESIAN_POINT('Ctrl Pts',(-0.00132303731134038,0.0137627584971618,
-0.00847711421478658));
#49375=CARTESIAN_POINT('Ctrl Pts',(-0.00190015089531529,0.0137355572567851,
-0.008802159380017));
#49376=CARTESIAN_POINT('Ctrl Pts',(-0.00220700152299049,0.0137210943886169,
-0.00897498551986764));
#49377=CARTESIAN_POINT('Ctrl Pts',(-0.00248978451650191,0.0137066315204487,
-0.00918980096997239));
#49378=CARTESIAN_POINT('Ctrl Pts',(-0.00273792804685609,0.0136921686522805,
-0.00943794641994652));
#49379=CARTESIAN_POINT('Ctrl Pts',(-0.0032133888562143,0.0136644567591069,
-0.00991341090743431));
#49380=CARTESIAN_POINT('Ctrl Pts',(-0.00356314378027725,0.0136367448659333,
-0.0105169991745023));
#49381=CARTESIAN_POINT('Ctrl Pts',(-0.00373869397446481,0.0136090329727596,
-0.0111686038808494));
#49382=CARTESIAN_POINT('Ctrl Pts',(-0.00382707773856266,0.0135950809435961,
-0.0114966654755253));
#49383=CARTESIAN_POINT('Ctrl Pts',(-0.00387200014747813,0.0135811289144327,
-0.0118364022358235));
#49384=CARTESIAN_POINT('Ctrl Pts',(-0.00387199999999964,0.0135671768852691,
-0.0121758549687856));
#49385=CARTESIAN_POINT('',(-0.003716429273515,0.0135218273791635,-0.0132634579329233));
#49386=CARTESIAN_POINT('Ctrl Pts',(-0.00387199984773757,0.0135691082707264,
-0.0121769391595942));
#49387=CARTESIAN_POINT('Ctrl Pts',(-0.00387189688840871,0.013553594427274,
-0.012544070944243));
#49388=CARTESIAN_POINT('Ctrl Pts',(-0.00381923731567736,0.013537090597348,
-0.0129110808850903));
#49389=CARTESIAN_POINT('Ctrl Pts',(-0.00371613325532325,0.013521920367515,
-0.0132633907013998));
#49390=CARTESIAN_POINT('',(-0.001845911937833,0.0135212256101277,-0.00877217981253542));
#49391=CARTESIAN_POINT('Origin',(0.,0.0135212256101277,-0.0121758532865581));
#49392=CARTESIAN_POINT('Ctrl Pts',(-0.00184591193783652,0.0135212256101277,
-0.00877217981253733));
#49393=CARTESIAN_POINT('Ctrl Pts',(-0.00124967671895911,0.0135491075912296,
-0.00844882396871596));
#49394=CARTESIAN_POINT('Ctrl Pts',(-0.000566623170632383,0.0135769895723315,
-0.0082859973652041));
#49395=CARTESIAN_POINT('Ctrl Pts',(0.000273039296966733,0.0136115349745585,
-0.00831009505947237));
#49396=CARTESIAN_POINT('Ctrl Pts',(0.000434650783267868,0.0136181983956836,
-0.00832492201216256));
#49397=CARTESIAN_POINT('Ctrl Pts',(0.00125539759212987,0.0136523856215694,
-0.00845247702085292));
#49398=CARTESIAN_POINT('Ctrl Pts',(0.00189000029279552,0.0136799094263301,
-0.00873076549636361));
#49399=CARTESIAN_POINT('Ctrl Pts',(0.00254715434705814,0.0137144548285571,
-0.00925462620708204));
#49400=CARTESIAN_POINT('Ctrl Pts',(0.00267361409669593,0.0137214764260234,
-0.0093699152669625));
#49401=CARTESIAN_POINT('Ctrl Pts',(0.00325663696424368,0.0137561008155063,
-0.00997661268728381));
#49402=CARTESIAN_POINT('Ctrl Pts',(0.00359322573364207,0.0137837036075229,
-0.0105846386258012));
#49403=CARTESIAN_POINT('Ctrl Pts',(0.00379719867837587,0.0138182490097499,
-0.0113998457298512));
#49404=CARTESIAN_POINT('Ctrl Pts',(0.00382743978479439,0.0138251916199603,
-0.0115663016482717));
#49405=CARTESIAN_POINT('Ctrl Pts',(0.00392323031147953,0.0138597271111741,
-0.0124000735232294));
#49406=CARTESIAN_POINT('Ctrl Pts',(0.00382254929095312,0.0138873199921774,
-0.0130874600833825));
#49407=CARTESIAN_POINT('Ctrl Pts',(0.00349085943066387,0.0139218653944044,
-0.0138595656610514));
#49408=CARTESIAN_POINT('Ctrl Pts',(0.00341393321808629,0.0139288179156281,
-0.0140105164085618));
#49409=CARTESIAN_POINT('Ctrl Pts',(0.0029846834402559,0.0139633633178551,
-0.0147319556112248));
#49410=CARTESIAN_POINT('Ctrl Pts',(0.00248800000162184,0.0139909561988584,
-0.0152176908676159));
#49411=CARTESIAN_POINT('Ctrl Pts',(0.00175621105354843,0.0140255016010854,
-0.0156308077414003));
#49412=CARTESIAN_POINT('Ctrl Pts',(0.00160353389092322,0.0140324541223091,
-0.0157042536173573));
#49413=CARTESIAN_POINT('Ctrl Pts',(0.000880174584334333,0.0140645449262985,
-0.0159956525091302));
#49414=CARTESIAN_POINT('Ctrl Pts',(0.000257583798528075,0.0140896832090642,
-0.0160873939728307));
#49415=CARTESIAN_POINT('Ctrl Pts',(-0.000351540291350107,0.0141148214918298,
-0.0160318620292294));
#49416=CARTESIAN_POINT('Origin',(0.,0.0118503152635658,-0.0121758532865581));
#49417=CARTESIAN_POINT('',(-0.0038721948279186,0.0143506728583483,-0.0121769419744163));
#49418=CARTESIAN_POINT('Ctrl Pts',(-0.000351540291350108,0.0141148214918298,
-0.0160318620292294));
#49419=CARTESIAN_POINT('Ctrl Pts',(-0.000579483589373538,0.0141242286112912,
-0.0160110811496345));
#49420=CARTESIAN_POINT('Ctrl Pts',(-0.000805485184122002,0.0141336357307525,
-0.0159700381770124));
#49421=CARTESIAN_POINT('Ctrl Pts',(-0.00102592211344818,0.0141430428502138,
-0.0159094665253843));
#49422=CARTESIAN_POINT('Ctrl Pts',(-0.00167088713486345,0.0141705666549745,
-0.0157322430596569));
#49423=CARTESIAN_POINT('Ctrl Pts',(-0.00226971427169042,0.0141980904597352,
-0.0153835001696018));
#49424=CARTESIAN_POINT('Ctrl Pts',(-0.00274234814416526,0.0142256142644959,
-0.0149093328742253));
#49425=CARTESIAN_POINT('Ctrl Pts',(-0.00286292176508331,0.0142326358619622,
-0.0147883680618112));
#49426=CARTESIAN_POINT('Ctrl Pts',(-0.00297542408952281,0.0142396574594285,
-0.0146594671455982));
#49427=CARTESIAN_POINT('Ctrl Pts',(-0.00307887154314382,0.0142466790568948,
-0.0145238170896903));
#49428=CARTESIAN_POINT('Ctrl Pts',(-0.00348964985403048,0.0142745610379969,
-0.0139851658335498));
#49429=CARTESIAN_POINT('Ctrl Pts',(-0.0037560121468941,0.0143024430190989,
-0.0133356522401737));
#49430=CARTESIAN_POINT('Ctrl Pts',(-0.00384129369772598,0.014330325000201,
-0.0126625222991433));
#49431=CARTESIAN_POINT('Ctrl Pts',(-0.0038616748494561,0.0143369884213259,
-0.0125016532327578));
#49432=CARTESIAN_POINT('Ctrl Pts',(-0.0038719340412436,0.0143436518424509,
-0.0123395196245888));
#49433=CARTESIAN_POINT('Ctrl Pts',(-0.00387199968253043,0.0143503152635758,
-0.012177421242004));
#49434=CARTESIAN_POINT('',(0.00380878994044106,0.0148791457076089,-0.0128757686928533));
#49435=CARTESIAN_POINT('Ctrl Pts',(-0.0038719999999991,0.0143503793522163,
-0.0121758559200756));
#49436=CARTESIAN_POINT('Ctrl Pts',(-0.00387200045770963,0.0143780325348381,
-0.01150289470167));
#49437=CARTESIAN_POINT('Ctrl Pts',(-0.00369222349743829,0.01440568571746,
-0.0108293876420033));
#49438=CARTESIAN_POINT('Ctrl Pts',(-0.00335670115622441,0.0144333389000819,
-0.0102458425747221));
#49439=CARTESIAN_POINT('Ctrl Pts',(-0.00315760406319418,0.0144497481450018,
-0.00989957017411986));
#49440=CARTESIAN_POINT('Ctrl Pts',(-0.00290472696423594,0.0144661573899216,
-0.00958484115308815));
#49441=CARTESIAN_POINT('Ctrl Pts',(-0.00261081926799486,0.0144825666348415,
-0.0093164815461461));
#49442=CARTESIAN_POINT('Ctrl Pts',(-0.00212574766486381,0.0145096488066976,
-0.00887357506081123));
#49443=CARTESIAN_POINT('Ctrl Pts',(-0.00152261847466415,0.0145367309785537,
-0.00855513870295691));
#49444=CARTESIAN_POINT('Ctrl Pts',(-0.000879918305563984,0.0145638131504098,
-0.00840516001137203));
#49445=CARTESIAN_POINT('Ctrl Pts',(-0.000476945286284811,0.014580793672722,
-0.00831112336865555));
#49446=CARTESIAN_POINT('Ctrl Pts',(-5.91672300722142E-5,0.0145977741950343,
-0.00828244179970653));
#49447=CARTESIAN_POINT('Ctrl Pts',(0.000351165990502362,0.0146147547173465,
-0.00831981043836327));
#49448=CARTESIAN_POINT('Ctrl Pts',(0.00100560491726355,0.0146418368892026,
-0.00837940954111882));
#49449=CARTESIAN_POINT('Ctrl Pts',(0.00164751455549754,0.0146689190610587,
-0.00861024688705076));
#49450=CARTESIAN_POINT('Ctrl Pts',(0.00219154154443199,0.0146960012329149,
-0.00898374901836311));
#49451=CARTESIAN_POINT('Ctrl Pts',(0.0025326464777122,0.0147129817552271,
-0.00921793486239789));
#49452=CARTESIAN_POINT('Ctrl Pts',(0.00283541353171744,0.0147299622775394,
-0.00950706446100596));
#49453=CARTESIAN_POINT('Ctrl Pts',(0.00308438600525397,0.0147469427998516,
-0.00983513823115442));
#49454=CARTESIAN_POINT('Ctrl Pts',(0.00348984360037339,0.0147745959843294,
-0.0103694141692799));
#49455=CARTESIAN_POINT('Ctrl Pts',(0.00375432056697956,0.0148022491688071,
-0.0110133833702221));
#49456=CARTESIAN_POINT('Ctrl Pts',(0.0038403218868933,0.0148299023532849,
-0.0116815742104804));
#49457=CARTESIAN_POINT('Ctrl Pts',(0.00389135541229657,0.0148463118629755,
-0.0120780813135661));
#49458=CARTESIAN_POINT('Ctrl Pts',(0.00388043750613101,0.0148627213726661,
-0.0124825444984827));
#49459=CARTESIAN_POINT('Ctrl Pts',(0.00380829892483911,0.0148791308823567,
-0.0128753125770599));
#49460=CARTESIAN_POINT('',(0.00147252214094898,0.0148792256101277,-0.0085947832587012));
#49461=CARTESIAN_POINT('Origin',(0.,0.0148792256101377,-0.0121758532865581));
#49462=CARTESIAN_POINT('',(-0.00387344021111285,0.0145664623429172,-0.012175597920995));
#49463=CARTESIAN_POINT('Ctrl Pts',(0.0014725221409559,0.0148792256101304,
-0.00859478325869949));
#49464=CARTESIAN_POINT('Ctrl Pts',(0.000887378242150321,0.0148532194115101,
-0.00835417514568843));
#49465=CARTESIAN_POINT('Ctrl Pts',(0.000242176794320239,0.0148310402855,
-0.00826224698544157));
#49466=CARTESIAN_POINT('Ctrl Pts',(-0.00038679968741254,0.0148044058086255,
-0.00832508349183273));
#49467=CARTESIAN_POINT('Ctrl Pts',(-0.000994091281060047,0.0147786895944635,
-0.0083857536173681));
#49468=CARTESIAN_POINT('Ctrl Pts',(-0.00158890100584688,0.0147498679363824,
-0.00858900078255042));
#49469=CARTESIAN_POINT('Ctrl Pts',(-0.00210175235193759,0.0147243548334753,
-0.00892093623646652));
#49470=CARTESIAN_POINT('Ctrl Pts',(-0.00212006501122793,0.0147234438233658,
-0.00893278883453473));
#49471=CARTESIAN_POINT('Ctrl Pts',(-0.00213827499674151,0.0147225370317578,
-0.00894480592354508));
#49472=CARTESIAN_POINT('Ctrl Pts',(-0.00215638108303436,0.0147216347506687,
-0.00895698443036752));
#49473=CARTESIAN_POINT('Ctrl Pts',(-0.00268155337858154,0.0146954638254269,
-0.00931022556049541));
#49474=CARTESIAN_POINT('Ctrl Pts',(-0.00311665188306085,0.0146740956855631,
-0.00979568174368227));
#49475=CARTESIAN_POINT('Ctrl Pts',(-0.00341452495792785,0.0146477578505066,
-0.0103532822316314));
#49476=CARTESIAN_POINT('Ctrl Pts',(-0.00369210313818325,0.0146232144830668,
-0.0108728918970016));
#49477=CARTESIAN_POINT('Ctrl Pts',(-0.00385395922200843,0.0145957954793885,
-0.0114565046869531));
#49478=CARTESIAN_POINT('Ctrl Pts',(-0.00387330707293454,0.0145710179582555,
-0.012045887858781));
#49479=CARTESIAN_POINT('Ctrl Pts',(-0.00387472167474202,0.0145692063706888,
-0.0120889801124556));
#49480=CARTESIAN_POINT('Ctrl Pts',(-0.00387537557451555,0.0145674089036423,
-0.012132109253815));
#49481=CARTESIAN_POINT('Ctrl Pts',(-0.00387528217137323,0.0145656277134538,
-0.0121752548237611));
#49482=CARTESIAN_POINT('Ctrl Pts',(-0.00387199999997852,0.0145671149317227,
-0.0121758661854451));
#49483=CARTESIAN_POINT('Ctrl Pts',(-0.00387199775389951,0.0145394030373481,
-0.0128500962879766));
#49484=CARTESIAN_POINT('Ctrl Pts',(-0.0036915722611453,0.0145116911429736,
-0.0135246572134559));
#49485=CARTESIAN_POINT('Ctrl Pts',(-0.00318550729473349,0.0144700270344287,
-0.0144029950422947));
#49486=CARTESIAN_POINT('Ctrl Pts',(-0.00297729196260053,0.0144560748202584,
-0.0146743978690617));
#49487=CARTESIAN_POINT('Ctrl Pts',(-0.00227184049541597,0.0144149583852686,
-0.0153798445279271));
#49488=CARTESIAN_POINT('Ctrl Pts',(-0.00168184678885426,0.0143877941644492,
-0.0157257004608036));
#49489=CARTESIAN_POINT('Ctrl Pts',(-0.000818093438899106,0.0143509604122953,
-0.0159677606078325));
#49490=CARTESIAN_POINT('Ctrl Pts',(-0.000585642423977778,0.0143412908809608,
-0.0160105196678911));
#49491=CARTESIAN_POINT('Ctrl Pts',(-0.000351540291350112,0.0143316213496264,
-0.0160318620292294));
#49492=CARTESIAN_POINT('Origin',(0.,0.0135212256101277,-0.0121758532865581));
#49493=CARTESIAN_POINT('',(-0.00441705924701761,0.0148779965858899,-0.0126490161932378));
#49494=CARTESIAN_POINT('Ctrl Pts',(-0.00444199982066862,0.0138992441597151,
-0.0121771154988945));
#49495=CARTESIAN_POINT('Ctrl Pts',(-0.00444202564285501,0.0139026434699815,
-0.0120862416070427));
#49496=CARTESIAN_POINT('Ctrl Pts',(-0.00443926284757712,0.0139059652244875,
-0.0119953857450405));
#49497=CARTESIAN_POINT('Ctrl Pts',(-0.00442784020811473,0.0139126423178769,
-0.0118086274885908));
#49498=CARTESIAN_POINT('Ctrl Pts',(-0.00441884605653583,0.0139159862346956,
-0.011712793506025));
#49499=CARTESIAN_POINT('Ctrl Pts',(-0.00436012104913382,0.0139318211304826,
-0.0112494584350861));
#49500=CARTESIAN_POINT('Ctrl Pts',(-0.00426762388218305,0.0139429719947748,
-0.0108889008820107));
#49501=CARTESIAN_POINT('Ctrl Pts',(-0.00408183008368174,0.0139587528637333,
-0.0104185152039224));
#49502=CARTESIAN_POINT('Ctrl Pts',(-0.00402656448691405,0.0139630294214672,
-0.0102953347732247));
#49503=CARTESIAN_POINT('Ctrl Pts',(-0.0039190876339132,0.0139709582836448,
-0.0100823251324102));
#49504=CARTESIAN_POINT('Ctrl Pts',(-0.00386917138242235,0.0139745238664448,
-0.00999144956897392));
#49505=CARTESIAN_POINT('Ctrl Pts',(-0.0037589689820606,0.0139823260620285,
-0.00980646792407794));
#49506=CARTESIAN_POINT('Ctrl Pts',(-0.00369821953128187,0.0139865846864293,
-0.00971272431953164));
#49507=CARTESIAN_POINT('Ctrl Pts',(-0.00345694603367115,0.014003057015773,
-0.00936948810311859));
#49508=CARTESIAN_POINT('Ctrl Pts',(-0.00325417807693909,0.014015993488214,
-0.00913669352427505));
#49509=CARTESIAN_POINT('Ctrl Pts',(-0.00286690602984965,0.0140373522192455,
-0.00877566206955802));
#49510=CARTESIAN_POINT('Ctrl Pts',(-0.00269376401373504,0.0140460078826927,
-0.00863691273066231));
#49511=CARTESIAN_POINT('Ctrl Pts',(-0.00238734867400198,0.0140597165348944,
-0.0084269345529207));
#49512=CARTESIAN_POINT('Ctrl Pts',(-0.00225950732541166,0.0140650257412601,
-0.00834852307781464));
#49513=CARTESIAN_POINT('Ctrl Pts',(-0.00180398266701824,0.0140826920725418,
-0.00809992200172164));
#49514=CARTESIAN_POINT('Ctrl Pts',(-0.00145927492313164,0.0140937984255215,
-0.00796419217128511));
#49515=CARTESIAN_POINT('Ctrl Pts',(-0.000957875691113172,0.0141097294880842,
-0.00783581957683498));
#49516=CARTESIAN_POINT('Ctrl Pts',(-0.00081225663396107,0.0141143537888474,
-0.00780622462977062));
#49517=CARTESIAN_POINT('Ctrl Pts',(-0.000557372889022838,0.0141227966525157,
-0.00776760590496824));
#49518=CARTESIAN_POINT('Ctrl Pts',(-0.000448748702513778,0.0141265036555715,
-0.00775522758600577));
#49519=CARTESIAN_POINT('Ctrl Pts',(-0.000240635274618488,0.0141339827762971,
-0.00773926144347405));
#49520=CARTESIAN_POINT('Ctrl Pts',(-0.00014126741769445,0.0141377235338807,
-0.00773498711422376));
#49521=CARTESIAN_POINT('Ctrl Pts',(0.000306994394699704,0.0141551135397262,
-0.00773076373155874));
#49522=CARTESIAN_POINT('Ctrl Pts',(0.000655010087065435,0.0141699083735277,
-0.00776858196043291));
#49523=CARTESIAN_POINT('Ctrl Pts',(0.00120088270129325,0.0141924504912556,
-0.00789404729244587));
#49524=CARTESIAN_POINT('Ctrl Pts',(0.0014031188511572,0.0142006717415967,
-0.00795598930669396));
#49525=CARTESIAN_POINT('Ctrl Pts',(0.0017389154139472,0.0142139322248016,
-0.00808566373784058));
#49526=CARTESIAN_POINT('Ctrl Pts',(0.00187486434873533,0.0142191892410764,
-0.00814616775676237));
#49527=CARTESIAN_POINT('Ctrl Pts',(0.00224729365688353,0.0142333740904071,
-0.00833485374749599));
#49528=CARTESIAN_POINT('Ctrl Pts',(0.00247554526504795,0.0142417772933865,
-0.00847784133140785));
#49529=CARTESIAN_POINT('Ctrl Pts',(0.00290080912554325,0.0142581730502546,
-0.00880136355572665));
#49530=CARTESIAN_POINT('Ctrl Pts',(0.00309728882477237,0.014266149521508,
-0.00898075391918834));
#49531=CARTESIAN_POINT('Ctrl Pts',(0.00334346015629937,0.0142782658930626,
-0.00924968594702028));
#49532=CARTESIAN_POINT('Ctrl Pts',(0.00340789540087553,0.0142816775959886,
-0.00932498854984708));
#49533=CARTESIAN_POINT('Ctrl Pts',(0.0035390771685509,0.0142892904191578,
-0.00948910385116271));
#49534=CARTESIAN_POINT('Ctrl Pts',(0.00360511680304918,0.0142935235954553,
-0.00957838917469358));
#49535=CARTESIAN_POINT('Ctrl Pts',(0.00384118729230714,0.0143099517519287,
-0.00992392484989375));
#49536=CARTESIAN_POINT('Ctrl Pts',(0.00398780770180776,0.0143228737041738,
-0.0101951219230348));
#49537=CARTESIAN_POINT('Ctrl Pts',(0.00416806792381943,0.0143419226672198,
-0.0106313051000987));
#49538=CARTESIAN_POINT('Ctrl Pts',(0.00422240145574149,0.0143484143021054,
-0.0107866986366084));
#49539=CARTESIAN_POINT('Ctrl Pts',(0.00431078430291874,0.0143605282374881,
-0.0110931060617778));
#49540=CARTESIAN_POINT('Ctrl Pts',(0.00434581377783233,0.0143661717611491,
-0.0112435922783342));
#49541=CARTESIAN_POINT('Ctrl Pts',(0.00440497242788833,0.0143779803658016,
-0.0115751502407589));
#49542=CARTESIAN_POINT('Ctrl Pts',(0.00442592101926712,0.0143840405180869,
-0.0117565016923853));
#49543=CARTESIAN_POINT('Ctrl Pts',(0.0044485050283149,0.0143975713436589,
-0.0121787980643437));
#49544=CARTESIAN_POINT('Ctrl Pts',(0.00444182285338998,0.0144048440842986,
-0.0124196075199902));
#49545=CARTESIAN_POINT('Ctrl Pts',(0.00439504372400568,0.0144181251602001,
-0.0128474188210095));
#49546=CARTESIAN_POINT('Ctrl Pts',(0.00436232903356552,0.0144240730846339,
-0.0130346240245222));
#49547=CARTESIAN_POINT('Ctrl Pts',(0.00429620162246521,0.0144336162605868,
-0.0133082960703997));
#49548=CARTESIAN_POINT('Ctrl Pts',(0.00427190638161057,0.0144368417064606,
-0.013396751043192));
#49549=CARTESIAN_POINT('Ctrl Pts',(0.004206342556907,0.0144450367530583,
-0.0136094390137663));
#49550=CARTESIAN_POINT('Ctrl Pts',(0.00416229188503837,0.0144501295990971,
-0.0137327116651824));
#49551=CARTESIAN_POINT('Ctrl Pts',(0.00403434800258625,0.014463667204684,
-0.0140463091881702));
#49552=CARTESIAN_POINT('Ctrl Pts',(0.00394241718416269,0.0144722938544275,
-0.0142330150455762));
#49553=CARTESIAN_POINT('Ctrl Pts',(0.00370430753313148,0.0144916471115149,
-0.0146415583246631));
#49554=CARTESIAN_POINT('Ctrl Pts',(0.00355062992283893,0.0145022380231317,
-0.0148581371018604));
#49555=CARTESIAN_POINT('Ctrl Pts',(0.00328200221519045,0.0145176958856387,
-0.0151728415838315));
#49556=CARTESIAN_POINT('Ctrl Pts',(0.00317983554487372,0.0145230350650933,
-0.0152810308739914));
#49557=CARTESIAN_POINT('Ctrl Pts',(0.00291987917654451,0.0145354483168824,
-0.0155299978923077));
#49558=CARTESIAN_POINT('Ctrl Pts',(0.00275709835575286,0.0145422831631224,
-0.0156650361916866));
#49559=CARTESIAN_POINT('Ctrl Pts',(0.00230163247088849,0.0145597961086379,
-0.0159910277457426));
#49560=CARTESIAN_POINT('Ctrl Pts',(0.00199504193389812,0.0145699609360743,
-0.0161599265322212));
#49561=CARTESIAN_POINT('Ctrl Pts',(0.00157974383068174,0.0145848500268095,
-0.0163286431974242));
#49562=CARTESIAN_POINT('Ctrl Pts',(0.00148637580315657,0.0145882723180297,
-0.0163629693617686));
#49563=CARTESIAN_POINT('Ctrl Pts',(0.0012881695489773,0.0145958323980512,
-0.0164283728988262));
#49564=CARTESIAN_POINT('Ctrl Pts',(0.00118318067977982,0.0145999960508943,
-0.016458771058935));
#49565=CARTESIAN_POINT('Ctrl Pts',(0.000933170033887146,0.01461010917163,
-0.0165212639361954));
#49566=CARTESIAN_POINT('Ctrl Pts',(0.000787445823063148,0.0146161554287245,
-0.016550019072331));
#49567=CARTESIAN_POINT('Ctrl Pts',(0.000275234332457088,0.0146373873156637,
-0.0166246630399494));
#49568=CARTESIAN_POINT('Ctrl Pts',(-9.53581726507817E-5,0.0146525639350941,
-0.0166321559733303));
#49569=CARTESIAN_POINT('Ctrl Pts',(-0.00061167697770944,0.0146719322510565,
-0.0165780886136249));
#49570=CARTESIAN_POINT('Ctrl Pts',(-0.000759850829046054,0.0146773045740417,
-0.016554946334376));
#49571=CARTESIAN_POINT('Ctrl Pts',(-0.00112358278574679,0.0146900996218849,
-0.0164791151526359));
#49572=CARTESIAN_POINT('Ctrl Pts',(-0.00133690223515231,0.0146972419957619,
-0.0164176927757886));
#49573=CARTESIAN_POINT('Ctrl Pts',(-0.00183341324129367,0.0147137641533747,
-0.0162335308955262));
#49574=CARTESIAN_POINT('Ctrl Pts',(-0.00211014030225272,0.0147228682765576,
-0.0160967510559873));
#49575=CARTESIAN_POINT('Ctrl Pts',(-0.00246486977430493,0.014736588663987,
-0.015872911145969));
#49576=CARTESIAN_POINT('Ctrl Pts',(-0.00255697215138027,0.0147403681868445,
-0.0158098195212305));
#49577=CARTESIAN_POINT('Ctrl Pts',(-0.00272988663573368,0.0147480751647543,
-0.0156815398685845));
#49578=CARTESIAN_POINT('Ctrl Pts',(-0.00281098163028683,0.0147519752446657,
-0.0156168558138115));
#49579=CARTESIAN_POINT('Ctrl Pts',(-0.00299230489974038,0.0147612267332673,
-0.0154615368153484));
#49580=CARTESIAN_POINT('Ctrl Pts',(-0.00309081359260155,0.0147666543088073,
-0.0153690450639589));
#49581=CARTESIAN_POINT('Ctrl Pts',(-0.00345781174343217,0.014788035248714,
-0.0149915465128209));
#49582=CARTESIAN_POINT('Ctrl Pts',(-0.00369241921182423,0.0148041250738692,
-0.0146759947882948));
#49583=CARTESIAN_POINT('Ctrl Pts',(-0.00395640640981797,0.0148242677548495,
-0.0142010143467172));
#49584=CARTESIAN_POINT('Ctrl Pts',(-0.00402333154541086,0.0148296748123009,
-0.0140645663290976));
#49585=CARTESIAN_POINT('Ctrl Pts',(-0.00418065875611654,0.0148433397730415,
-0.0136972973811787));
#49586=CARTESIAN_POINT('Ctrl Pts',(-0.00425897224168211,0.0148511999675334,
-0.0134618803121984));
#49587=CARTESIAN_POINT('Ctrl Pts',(-0.00436286304922231,0.0148648375902373,
-0.0130327950468715));
#49588=CARTESIAN_POINT('Ctrl Pts',(-0.004396092120752,0.0148706917529315,
-0.0128416570437104));
#49589=CARTESIAN_POINT('Ctrl Pts',(-0.00441673296289603,0.0148767675448707,
-0.012648964197939));
#49590=CARTESIAN_POINT('',(-0.00278820502685331,0.0148792256101277,-0.0156337828301188));
#49591=CARTESIAN_POINT('Origin',(0.,0.0148792256101377,-0.0121758532865581));
#49592=CARTESIAN_POINT('Ctrl Pts',(-0.00278820502685448,0.0148792256101377,
-0.0156337828301179));
#49593=CARTESIAN_POINT('Ctrl Pts',(-0.00201147069505603,0.0148434782482309,
-0.0162600808911887));
#49594=CARTESIAN_POINT('Ctrl Pts',(-2.30099782061264E-5,0.0147719835244173,
-0.0169665420603791));
#49595=CARTESIAN_POINT('Ctrl Pts',(0.00297216531875188,0.0146647414386969,
-0.015933805333576));
#49596=CARTESIAN_POINT('Ctrl Pts',(0.00466732644442066,0.0145574993529764,
-0.0132576561457133));
#49597=CARTESIAN_POINT('Ctrl Pts',(0.00432221053072379,0.014450257267256,
-0.0101086911624707));
#49598=CARTESIAN_POINT('Ctrl Pts',(0.00208747382629606,0.0143430151815356,
-0.00786346571244169));
#49599=CARTESIAN_POINT('Ctrl Pts',(-0.00105984742215624,0.0142357730958152,
-0.00750330647444095));
#49600=CARTESIAN_POINT('Ctrl Pts',(-0.0037438236759896,0.0141285312769041,
-0.00918670830698344));
#49601=CARTESIAN_POINT('Ctrl Pts',(-0.00444200032332976,0.0140570368198998,
-0.0111780827837936));
#49602=CARTESIAN_POINT('Ctrl Pts',(-0.00444199999999725,0.0140212897248023,
-0.0121758555835873));
#49603=CARTESIAN_POINT('Origin',(0.,0.0137212256101277,-0.0121758532865581));
#49604=CARTESIAN_POINT('',(-0.0025,0.0139212256101277,-0.0121758532865581));
#49605=CARTESIAN_POINT('Origin',(0.,0.0139212256101377,-0.0121758532865581));
#49606=CARTESIAN_POINT('',(-0.002900000000005,0.0135212256101227,-0.0121758532865581));
#49607=CARTESIAN_POINT('',(-0.0027,0.0137212256101277,-0.0121758532865581));
#49608=CARTESIAN_POINT('Origin',(0.,0.0135212256101277,-0.0121758532865581));
#49609=CARTESIAN_POINT('Origin',(0.,0.0135212256101277,-0.0121758532865581));
#49610=CARTESIAN_POINT('',(-0.0025,0.0151212256101377,-0.0121758532865581));
#49611=CARTESIAN_POINT('',(-0.0025,0.0135212256101277,-0.0121758532865581));
#49612=CARTESIAN_POINT('Origin',(0.,0.0151212256101377,-0.0121758532865581));
#49613=CARTESIAN_POINT('Origin',(0.,0.0135212256101277,-0.0121758532865581));
#49614=CARTESIAN_POINT('',(-0.00371483287819128,0.013521225610129,-0.0132805663438727));
#49615=CARTESIAN_POINT('Ctrl Pts',(-0.0037148328777567,0.0135212256101303,
-0.0132805663459238));
#49616=CARTESIAN_POINT('Ctrl Pts',(-0.00367676010924277,0.0135212256101305,
-0.0134593107044183));
#49617=CARTESIAN_POINT('Ctrl Pts',(-0.00362588667618153,0.0135212256101307,
-0.0136344111414368));
#49618=CARTESIAN_POINT('Ctrl Pts',(-0.00356215531751432,0.0135212256101308,
-0.0138044431938857));
#49619=CARTESIAN_POINT('Ctrl Pts',(-0.00352036300244373,0.0135212256101308,
-0.0139159429838894));
#49620=CARTESIAN_POINT('Ctrl Pts',(-0.00347303710944158,0.0135212256101309,
-0.0140252648516543));
#49621=CARTESIAN_POINT('Ctrl Pts',(-0.0034205447519999,0.0135212256101335,
-0.0141322036001223));
#49622=CARTESIAN_POINT('Ctrl Pts',(-0.00336697272343145,0.0135212256101361,
-0.0142413418817163));
#49623=CARTESIAN_POINT('Ctrl Pts',(-0.00330801916308001,0.0135212256101311,
-0.0143479986131602));
#49624=CARTESIAN_POINT('Ctrl Pts',(-0.00324402262044731,0.0135212256101344,
-0.0144519391983276));
#49625=CARTESIAN_POINT('Ctrl Pts',(-0.00320932607863089,0.0135212256101362,
-0.0145082919122607));
#49626=CARTESIAN_POINT('Ctrl Pts',(-0.00317314634461811,0.0135212256101312,
-0.0145638459036323));
#49627=CARTESIAN_POINT('Ctrl Pts',(-0.00313553181154857,0.0135212256101312,
-0.0146185608267094));
#49628=CARTESIAN_POINT('Ctrl Pts',(-0.00312568654141207,0.0135212256101312,
-0.0146328819721347));
#49629=CARTESIAN_POINT('Ctrl Pts',(-0.00311574295633818,0.0135212256101312,
-0.0146471456214485));
#49630=CARTESIAN_POINT('Ctrl Pts',(-0.00310570188433775,0.0135212256101312,
-0.0146613510227781));
#49631=CARTESIAN_POINT('Ctrl Pts',(-0.00309590668589143,0.0135212256101312,
-0.0146752085795238));
#49632=CARTESIAN_POINT('Ctrl Pts',(-0.00308602434663422,0.0135212256101312,
-0.0146890027305733));
#49633=CARTESIAN_POINT('Ctrl Pts',(-0.00307605677284421,0.0135212256101312,
-0.0147027318404865));
#49634=CARTESIAN_POINT('Ctrl Pts',(-0.00300316097838175,0.0135212256101313,
-0.0148031368533285));
#49635=CARTESIAN_POINT('Ctrl Pts',(-0.00292569704568872,0.0135212256101363,
-0.0149000838514716));
#49636=CARTESIAN_POINT('Ctrl Pts',(-0.00284407294034953,0.0135212256101338,
-0.0149933598189867));
#49637=CARTESIAN_POINT('Ctrl Pts',(-0.00276104793101491,0.0135212256101313,
-0.0150882366699054));
#49638=CARTESIAN_POINT('Ctrl Pts',(-0.00267371826719912,0.0135212256101313,
-0.0151793160423849));
#49639=CARTESIAN_POINT('Ctrl Pts',(-0.00258246178724139,0.0135212256101313,
-0.0152663540581625));
#49640=CARTESIAN_POINT('Ctrl Pts',(-0.00243774910228737,0.0135212256101313,
-0.0154043771877208));
#49641=CARTESIAN_POINT('Ctrl Pts',(-0.00228317140345813,0.0135212256101313,
-0.015532250623269));
#49642=CARTESIAN_POINT('Ctrl Pts',(-0.00212002316546883,0.0135212256101312,
-0.0156488439511656));
#49643=CARTESIAN_POINT('Ctrl Pts',(-0.00208706339792013,0.0135212256101312,
-0.0156723985358339));
#49644=CARTESIAN_POINT('Ctrl Pts',(-0.00205375312855055,0.0135212256101312,
-0.0156954919643269));
#49645=CARTESIAN_POINT('Ctrl Pts',(-0.00202010203786124,0.0135212256101312,
-0.0157181136505389));
#49646=CARTESIAN_POINT('Ctrl Pts',(-0.0020052538477559,0.0135212256101312,
-0.0157280952318338));
#49647=CARTESIAN_POINT('Ctrl Pts',(-0.00199033775336458,0.0135212256101312,
-0.0157379859714015));
#49648=CARTESIAN_POINT('Ctrl Pts',(-0.00197535945581412,0.0135212256101312,
-0.0157477817383071));
#49649=CARTESIAN_POINT('Ctrl Pts',(-0.00186683699532327,0.0135212256101312,
-0.015818755139884));
#49650=CARTESIAN_POINT('Ctrl Pts',(-0.00175538512191969,0.0135212256101362,
-0.0158845295934832));
#49651=CARTESIAN_POINT('Ctrl Pts',(-0.00164139770383617,0.0135212256101336,
-0.0159448584383389));
#49652=CARTESIAN_POINT('Ctrl Pts',(-0.00152735310373093,0.013521225610131,
-0.0160052175472831));
#49653=CARTESIAN_POINT('Ctrl Pts',(-0.00141076975051351,0.0135212256101309,
-0.0160601262200838));
#49654=CARTESIAN_POINT('Ctrl Pts',(-0.00129200332480448,0.0135212256101308,
-0.0161093027019261));
#49655=CARTESIAN_POINT('Ctrl Pts',(-0.00111285742462027,0.0135212256101308,
-0.0161834799372428));
#49656=CARTESIAN_POINT('Ctrl Pts',(-0.000928748119590978,0.0135212256101306,
-0.0162446291259923));
#49657=CARTESIAN_POINT('Ctrl Pts',(-0.000740778709230239,0.0135212256101304,
-0.0162915858099064));
#49658=CARTESIAN_POINT('Ctrl Pts',(-0.00069400337526837,0.0135212256101304,
-0.0163032707674088));
#49659=CARTESIAN_POINT('Ctrl Pts',(-0.00064698849963088,0.0135212256101304,
-0.0163140755329016));
#49660=CARTESIAN_POINT('Ctrl Pts',(-0.000599754198781191,0.0135212256101303,
-0.0163240069284197));
#49661=CARTESIAN_POINT('Ctrl Pts',(-0.000571358594604591,0.0135212256101303,
-0.0163299773349036));
#49662=CARTESIAN_POINT('Ctrl Pts',(-0.000542883685759838,0.0135212256101303,
-0.016335632085061));
#49663=CARTESIAN_POINT('Ctrl Pts',(-0.000514333811540033,0.0135212256101303,
-0.0163409724716758));
#49664=CARTESIAN_POINT('Ctrl Pts',(-0.000497614725750705,0.0135212256101302,
-0.0163440998543492));
#49665=CARTESIAN_POINT('Ctrl Pts',(-0.000480871848590969,0.0135212256101352,
-0.0163471190178022));
#49666=CARTESIAN_POINT('Ctrl Pts',(-0.000464117417771817,0.0135212256101346,
-0.0163500284533313));
#49667=CARTESIAN_POINT('Ctrl Pts',(-0.000341217338960648,0.0135212256101301,
-0.0163713702619364));
#49668=CARTESIAN_POINT('Ctrl Pts',(-0.000217529147290246,0.0135212256101298,
-0.0163868437048162));
#49669=CARTESIAN_POINT('Ctrl Pts',(-9.3428659998974E-5,0.0135212256101295,
-0.0163966664507915));
#49670=CARTESIAN_POINT('Ctrl Pts',(3.36391484278545E-5,0.0135212256101292,
-0.0164067240648353));
#49671=CARTESIAN_POINT('Ctrl Pts',(0.000161139813868302,0.0135212256101295,
-0.0164108575969878));
#49672=CARTESIAN_POINT('Ctrl Pts',(0.000288690269230646,0.0135212256101296,
-0.0164092501650054));
#49673=CARTESIAN_POINT('Ctrl Pts',(0.000532010107936883,0.0135212256101298,
-0.0164061837699105));
#49674=CARTESIAN_POINT('Ctrl Pts',(0.000775513572144928,0.0135212256101301,
-0.0163822632742277));
#49675=CARTESIAN_POINT('Ctrl Pts',(0.00101661218976315,0.0135212256101302,
-0.0163382677180292));
#49676=CARTESIAN_POINT('Ctrl Pts',(0.00104574194951984,0.0135212256101303,
-0.0163329521339122));
#49677=CARTESIAN_POINT('Ctrl Pts',(0.00107483656722365,0.0135212256101353,
-0.0163273427497234));
#49678=CARTESIAN_POINT('Ctrl Pts',(0.00110389140778561,0.0135212256101353,
-0.0163214403265222));
#49679=CARTESIAN_POINT('Ctrl Pts',(0.00112687781898231,0.0135212256101353,
-0.0163167706906153));
#49680=CARTESIAN_POINT('Ctrl Pts',(0.00114984177385114,0.0135212256101303,
-0.0163119170173606));
#49681=CARTESIAN_POINT('Ctrl Pts',(0.00117275806504747,0.0135212256101303,
-0.0163068849107322));
#49682=CARTESIAN_POINT('Ctrl Pts',(0.00130317602529154,0.0135212256101305,
-0.0162782468961171));
#49683=CARTESIAN_POINT('Ctrl Pts',(0.00143220650179616,0.0135212256101355,
-0.0162438036971463));
#49684=CARTESIAN_POINT('Ctrl Pts',(0.00155943569693481,0.0135212256101356,
-0.0162037234389758));
#49685=CARTESIAN_POINT('Ctrl Pts',(0.00168729814890097,0.0135212256101357,
-0.0161634436896657));
#49686=CARTESIAN_POINT('Ctrl Pts',(0.00181334218941698,0.0135212256101308,
-0.016117470513265));
#49687=CARTESIAN_POINT('Ctrl Pts',(0.00193714485169985,0.0135212256101309,
-0.0160659222475803));
#49688=CARTESIAN_POINT('Ctrl Pts',(0.00199197341364183,0.0135212256101309,
-0.0160430930351387));
#49689=CARTESIAN_POINT('Ctrl Pts',(0.00204636224868705,0.0135212256101359,
-0.0160191696812025));
#49690=CARTESIAN_POINT('Ctrl Pts',(0.00210027376306881,0.0135212256101328,
-0.0159941592988056));
#49691=CARTESIAN_POINT('Ctrl Pts',(0.00213093281696214,0.013521225610131,
-0.0159799360911923));
#49692=CARTESIAN_POINT('Ctrl Pts',(0.00216143748795381,0.013521225610131,
-0.0159653612919411));
#49693=CARTESIAN_POINT('Ctrl Pts',(0.00219178074621081,0.013521225610131,
-0.0159504359356592));
#49694=CARTESIAN_POINT('Ctrl Pts',(0.00221206061632124,0.013521225610131,
-0.0159404605966833));
#49695=CARTESIAN_POINT('Ctrl Pts',(0.00223225959097951,0.013521225610131,
-0.0159303329738333));
#49696=CARTESIAN_POINT('Ctrl Pts',(0.00225237355325245,0.013521225610131,
-0.0159200548931265));
#49697=CARTESIAN_POINT('Ctrl Pts',(0.00237320353572851,0.0135212256101311,
-0.0158583116972888));
#49698=CARTESIAN_POINT('Ctrl Pts',(0.00249099215410104,0.0135212256101311,
-0.0157911304018793));
#49699=CARTESIAN_POINT('Ctrl Pts',(0.00260531366703308,0.0135212256101312,
-0.0157186451039207));
#49700=CARTESIAN_POINT('Ctrl Pts',(0.00271786118642715,0.0135212256101312,
-0.015647284602572));
#49701=CARTESIAN_POINT('Ctrl Pts',(0.00282704914459482,0.0135212256101363,
-0.015570783150034));
#49702=CARTESIAN_POINT('Ctrl Pts',(0.00293245440604282,0.0135212256101363,
-0.0154892218352429));
#49703=CARTESIAN_POINT('Ctrl Pts',(0.00300373533197715,0.0135212256101363,
-0.0154340655180073));
#49704=CARTESIAN_POINT('Ctrl Pts',(0.00307328599312713,0.0135212256101313,
-0.0153765942559097));
#49705=CARTESIAN_POINT('Ctrl Pts',(0.00314096832203064,0.0135212256101277,
-0.0153168216085888));
#49706=CARTESIAN_POINT('Ctrl Pts',(0.00444614404405592,0.0135212256101274,
-0.0121732434012118));
#49707=CARTESIAN_POINT('Ctrl Pts',(0.00443886810540444,0.0135212256101255,
-0.0120407103896413));
#49708=CARTESIAN_POINT('Ctrl Pts',(0.00442548803232603,0.0135212256101254,
-0.0119089346953794));
#49709=CARTESIAN_POINT('Ctrl Pts',(0.00440586757070844,0.0135212256101253,
-0.0117782950810129));
#49710=CARTESIAN_POINT('Ctrl Pts',(0.00439482636005699,0.0135212256101252,
-0.0117047789971533));
#49711=CARTESIAN_POINT('Ctrl Pts',(0.00438180805572112,0.0135212256101251,
-0.0116316227160819));
#49712=CARTESIAN_POINT('Ctrl Pts',(0.00436678116022483,0.013521225610125,
-0.011558894860445));
#49713=CARTESIAN_POINT('Ctrl Pts',(0.00429880769955738,0.0135212256101248,
-0.011229913798736));
#49714=CARTESIAN_POINT('Ctrl Pts',(0.00418987598555604,0.0135212256101246,
-0.0109096134480047));
#49715=CARTESIAN_POINT('Ctrl Pts',(0.00404445376166765,0.0135212256101244,
-0.0106037286146905));
#49716=CARTESIAN_POINT('Ctrl Pts',(0.00403582379204659,0.0135212256101244,
-0.0105855761153788));
#49717=CARTESIAN_POINT('Ctrl Pts',(0.00402706483909659,0.0135212256101244,
-0.0105674747504207));
#49718=CARTESIAN_POINT('Ctrl Pts',(0.00401817766918596,0.0135212256101244,
-0.0105494258704874));
#49719=CARTESIAN_POINT('Ctrl Pts',(0.00401119004020987,0.0135212256101244,
-0.0105352347525414));
#49720=CARTESIAN_POINT('Ctrl Pts',(0.00400412394035098,0.0135212256101244,
-0.0105210777685657));
#49721=CARTESIAN_POINT('Ctrl Pts',(0.00399698403616598,0.0135212256101244,
-0.0105069637321066));
#49722=CARTESIAN_POINT('Ctrl Pts',(0.00381744654911037,0.0135212256101242,
-0.0101520571994109));
#49723=CARTESIAN_POINT('Ctrl Pts',(0.00359079765244732,0.0135212256101241,
-0.00982262213931191));
#49724=CARTESIAN_POINT('Ctrl Pts',(0.00332467018493774,0.0135212256101241,
-0.00952801515336511));
#49725=CARTESIAN_POINT('Ctrl Pts',(0.00327375278488671,0.0135212256101241,
-0.00947164884927159));
#49726=CARTESIAN_POINT('Ctrl Pts',(0.0032213815704452,0.013521225610119,
-0.00941656604383548));
#49727=CARTESIAN_POINT('Ctrl Pts',(0.0031675992986144,0.013521225610119,
-0.00936284615281305));
#49728=CARTESIAN_POINT('Ctrl Pts',(0.00313750849569358,0.013521225610119,
-0.00933279025151588));
#49729=CARTESIAN_POINT('Ctrl Pts',(0.0031069759402194,0.0135212256101241,
-0.00930316108343312));
#49730=CARTESIAN_POINT('Ctrl Pts',(0.00307600881182139,0.0135212256101241,
-0.00927397334107523));
#49731=CARTESIAN_POINT('Ctrl Pts',(0.00305592031613699,0.0135212256101241,
-0.00925503913998115));
#49732=CARTESIAN_POINT('Ctrl Pts',(0.0030356489406292,0.0135212256101191,
-0.00923629070985852));
#49733=CARTESIAN_POINT('Ctrl Pts',(0.00301519660291451,0.0135212256101191,
-0.00921773219655775));
#49734=CARTESIAN_POINT('Ctrl Pts',(0.00290572585389851,0.0135212256101191,
-0.00911839810673394));
#49735=CARTESIAN_POINT('Ctrl Pts',(0.00279161951354767,0.0135212256101191,
-0.00902499526771897));
#49736=CARTESIAN_POINT('Ctrl Pts',(0.00267329637337972,0.0135212256101191,
-0.00893802803368589));
#49737=CARTESIAN_POINT('Ctrl Pts',(0.00257075184570355,0.0135212256101192,
-0.00886265804329714));
#49738=CARTESIAN_POINT('Ctrl Pts',(0.00246503183794056,0.0135212256101242,
-0.00879211589896134));
#49739=CARTESIAN_POINT('Ctrl Pts',(0.00235636239577334,0.0135212256101242,
-0.00872675896201271));
#49740=CARTESIAN_POINT('Ctrl Pts',(0.00219814089042433,0.0135212256101243,
-0.00863159998500149));
#49741=CARTESIAN_POINT('Ctrl Pts',(0.00203366811371355,0.0135212256101244,
-0.00854742067631489));
#49742=CARTESIAN_POINT('Ctrl Pts',(0.00186357782707476,0.0135212256101245,
-0.00847552126255479));
#49743=CARTESIAN_POINT('Ctrl Pts',(0.00179024018558216,0.0135212256101246,
-0.00844452047153923));
#49744=CARTESIAN_POINT('Ctrl Pts',(0.00171585740388813,0.0135212256101246,
-0.00841580601568659));
#49745=CARTESIAN_POINT('Ctrl Pts',(0.00164053200032731,0.0135212256101247,
-0.00838938077384102));
#49746=CARTESIAN_POINT('Ctrl Pts',(0.0016227936715147,0.0135212256101247,
-0.00838315791134508));
#49747=CARTESIAN_POINT('Ctrl Pts',(0.00160501052496767,0.0135212256101247,
-0.00837706468038289));
#49748=CARTESIAN_POINT('Ctrl Pts',(0.00158719063949712,0.0135212256101247,
-0.00837110296172034));
#49749=CARTESIAN_POINT('Ctrl Pts',(0.00112804892776666,0.0135212256101251,
-0.00821749514442541));
#49750=CARTESIAN_POINT('Ctrl Pts',(0.000643190067065385,0.0135212256101255,
-0.00814977887709749));
#49751=CARTESIAN_POINT('Ctrl Pts',(0.000156630255982111,0.013521225610126,
-0.00816621136866286));
#49752=CARTESIAN_POINT('Ctrl Pts',(0.000132844566441299,0.0135212256101261,
-0.00816701467821259));
#49753=CARTESIAN_POINT('Ctrl Pts',(0.000109055105933201,0.0135212256101261,
-0.00816802124209177));
#49754=CARTESIAN_POINT('Ctrl Pts',(8.52648460987993E-5,0.0135212256101261,
-0.0081692315113233));
#49755=CARTESIAN_POINT('Ctrl Pts',(6.53964806939949E-5,0.0135212256101261,
-0.00817024226410605));
#49756=CARTESIAN_POINT('Ctrl Pts',(4.55369000206317E-5,0.0135212256101262,
-0.00817139463835654));
#49757=CARTESIAN_POINT('Ctrl Pts',(2.56914149112288E-5,0.0135212256101261,
-0.00817268824315978));
#49758=CARTESIAN_POINT('Ctrl Pts',(-0.000298296126733115,0.0135212256101251,
-0.00819380699323063));
#49759=CARTESIAN_POINT('Ctrl Pts',(-0.000618909869140803,0.013521225610125,
-0.00825239931907039));
#49760=CARTESIAN_POINT('Ctrl Pts',(-0.000928653071344667,0.0135212256101248,
-0.00834875706957382));
#49761=CARTESIAN_POINT('Ctrl Pts',(-0.000948935745052395,0.0135212256101248,
-0.00835506678936352));
#49762=CARTESIAN_POINT('Ctrl Pts',(-0.000969162136026976,0.0135212256101248,
-0.00836153633871243));
#49763=CARTESIAN_POINT('Ctrl Pts',(-0.000989328103931621,0.0135212256101248,
-0.00836816498528667));
#49764=CARTESIAN_POINT('Ctrl Pts',(-0.00110526038790483,0.0135212256101247,
-0.00840627246124005));
#49765=CARTESIAN_POINT('Ctrl Pts',(-0.00121922018951225,0.0135212256101196,
-0.00844964141738153));
#49766=CARTESIAN_POINT('Ctrl Pts',(-0.00133080618113665,0.013521225610122,
-0.00849828346020436));
#49767=CARTESIAN_POINT('Ctrl Pts',(-0.00143947616796051,0.0135212256101244,
-0.0085456543718725));
#49768=CARTESIAN_POINT('Ctrl Pts',(-0.00154589536550546,0.0135212256101244,
-0.00859802668055264));
#49769=CARTESIAN_POINT('Ctrl Pts',(-0.00164966624456178,0.0135212256101243,
-0.0086554518957699));
#49770=CARTESIAN_POINT('Ctrl Pts',(-0.00171620850601353,0.0135212256101243,
-0.0086922753641616));
#49771=CARTESIAN_POINT('Ctrl Pts',(-0.00178166123650336,0.0135212256101192,
-0.00873117735060907));
#49772=CARTESIAN_POINT('Ctrl Pts',(-0.00184591193783782,0.0135212256101219,
-0.00877217981252655));
#49773=CARTESIAN_POINT('Ctrl Pts',(-0.00371483287808303,0.0135212256101277,
-0.01328056634437));
#49774=CARTESIAN_POINT('Ctrl Pts',(-0.00371549183366996,0.0135212256101277,
-0.0132774726740512));
#49775=CARTESIAN_POINT('Ctrl Pts',(-0.0037161468930533,0.0135212256101277,
-0.0132743781740399));
#49776=CARTESIAN_POINT('Ctrl Pts',(-0.00371731615019988,0.0135212256101277,
-0.0132688200925666));
#49777=CARTESIAN_POINT('Ctrl Pts',(-0.003717831777219,0.0135212256101277,
-0.0132663568120799));
#49778=CARTESIAN_POINT('Ctrl Pts',(-0.00371834493906906,0.0135212256101277,
-0.0132638930180542));
#49779=CARTESIAN_POINT('Origin',(0.,0.0153212256101277,-0.0121758532865581));
#49780=CARTESIAN_POINT('',(-0.00290000000001,0.0155212256101377,-0.0121758532865581));
#49781=CARTESIAN_POINT('',(-0.0027,0.0153212256101277,-0.0121758532865581));
#49782=CARTESIAN_POINT('Origin',(0.,0.0155212256101377,-0.0121758532865581));
#49783=CARTESIAN_POINT('Origin',(0.,0.0155212256101277,-0.0121758532865581));
#49784=CARTESIAN_POINT('',(-0.0038,0.0155212256101277,-0.0121758532865581));
#49785=CARTESIAN_POINT('Origin',(0.,0.0155212256101377,-0.0121758532865581));
#49786=CARTESIAN_POINT('Origin',(4.78424556569738E-19,0.0148792256101277,
-0.0121758532865581));
#49787=CARTESIAN_POINT('',(-0.00442435797140522,0.0148792256101377,-0.0125713536543859));
#49788=CARTESIAN_POINT('',(-0.00444200000001,0.0148792256101377,-0.0121758532865581));
#49789=CARTESIAN_POINT('Origin',(0.,0.0148792256101377,-0.0121758532865581));
#49790=CARTESIAN_POINT('Ctrl Pts',(-0.00442435797140521,0.0148792256101308,
-0.0125713536543859));
#49791=CARTESIAN_POINT('Ctrl Pts',(-0.00442800643686139,0.0148792260236933,
-0.0124648769960618));
#49792=CARTESIAN_POINT('Ctrl Pts',(-0.00442766428860729,0.0148792256101345,
-0.012358442139106));
#49793=CARTESIAN_POINT('Ctrl Pts',(-0.00442322426732517,0.0148792256101344,
-0.0122522393837103));
#49794=CARTESIAN_POINT('Ctrl Pts',(-0.00442009298055464,0.0148792256101343,
-0.0121773408051147));
#49795=CARTESIAN_POINT('Ctrl Pts',(-0.00441492275573164,0.0148792256101349,
-0.012102557690367));
#49796=CARTESIAN_POINT('Ctrl Pts',(-0.00440766855611385,0.014879225610135,
-0.0120279578270332));
#49797=CARTESIAN_POINT('Ctrl Pts',(-0.00439351054235581,0.0148792256101351,
-0.0118823613522907));
#49798=CARTESIAN_POINT('Ctrl Pts',(-0.00437141830531153,0.0148792256101352,
-0.0117374609477969));
#49799=CARTESIAN_POINT('Ctrl Pts',(-0.00434171523037098,0.0148792256101353,
-0.0115937591489407));
#49800=CARTESIAN_POINT('Ctrl Pts',(-0.00433640963489609,0.0148792256101354,
-0.0115680909777069));
#49801=CARTESIAN_POINT('Ctrl Pts',(-0.00433086104162323,0.0148792256101354,
-0.0115424611293754));
#49802=CARTESIAN_POINT('Ctrl Pts',(-0.00432507107819976,0.0148792256101354,
-0.0115168725829161));
#49803=CARTESIAN_POINT('Ctrl Pts',(-0.00432033646974495,0.0148792256101354,
-0.011495948141853));
#49804=CARTESIAN_POINT('Ctrl Pts',(-0.00431544270971432,0.0148792256101354,
-0.0114750612571913));
#49805=CARTESIAN_POINT('Ctrl Pts',(-0.00431039114734557,0.0148792256101355,
-0.0114542136188716));
#49806=CARTESIAN_POINT('Ctrl Pts',(-0.00423477824437842,0.0148792256101357,
-0.011142161556897));
#49807=CARTESIAN_POINT('Ctrl Pts',(-0.00412393664690842,0.0148792256101358,
-0.0108388232708057));
#49808=CARTESIAN_POINT('Ctrl Pts',(-0.0039813631737944,0.014879225610136,
-0.0105495620737052));
#49809=CARTESIAN_POINT('Ctrl Pts',(-0.00396120669884738,0.014879225610136,
-0.0105086674672601));
#49810=CARTESIAN_POINT('Ctrl Pts',(-0.00394040419837136,0.0148792256101361,
-0.010468038341568));
#49811=CARTESIAN_POINT('Ctrl Pts',(-0.00391899916438485,0.0148792256101361,
-0.0104277578853243));
#49812=CARTESIAN_POINT('Ctrl Pts',(-0.00364785767429892,0.0148792256101363,
-0.0099175179607283));
#49813=CARTESIAN_POINT('Ctrl Pts',(-0.00328050367389714,0.0148792256101364,
-0.00946181130830208));
#49814=CARTESIAN_POINT('Ctrl Pts',(-0.0028374264715703,0.0148792256101363,
-0.00909769299540765));
#49815=CARTESIAN_POINT('Ctrl Pts',(-0.0026578942354509,0.0148792256101363,
-0.00895015442970699));
#49816=CARTESIAN_POINT('Ctrl Pts',(-0.00246696490726739,0.0148792256101362,
-0.00881866982220281));
#49817=CARTESIAN_POINT('Ctrl Pts',(-0.00226578756927449,0.0148792256101361,
-0.00870553397651577));
#49818=CARTESIAN_POINT('Ctrl Pts',(-0.0022596861691341,0.0148792256101361,
-0.00870210273981861));
#49819=CARTESIAN_POINT('Ctrl Pts',(-0.00225357532131785,0.0148792256101361,
-0.00869868842155052));
#49820=CARTESIAN_POINT('Ctrl Pts',(-0.00224745505410032,0.0148792256101361,
-0.00869529109370495));
#49821=CARTESIAN_POINT('Ctrl Pts',(-0.00204000448908894,0.014879225610136,
-0.00858013638623183));
#49822=CARTESIAN_POINT('Ctrl Pts',(-0.0018217385611798,0.0148792256101359,
-0.00848445099112787));
#49823=CARTESIAN_POINT('Ctrl Pts',(-0.00159542878803322,0.0148792256101357,
-0.00840845967616131));
#49824=CARTESIAN_POINT('Ctrl Pts',(-0.00157798612369806,0.0148792256101357,
-0.00840260269976599));
#49825=CARTESIAN_POINT('Ctrl Pts',(-0.00156049566425499,0.0148792256101357,
-0.00839686301748051));
#49826=CARTESIAN_POINT('Ctrl Pts',(-0.0015429586822898,0.0148792256101356,
-0.0083912408836659));
#49827=CARTESIAN_POINT('Ctrl Pts',(-0.00152548865319278,0.0148792256101356,
-0.00838564021409097));
#49828=CARTESIAN_POINT('Ctrl Pts',(-0.00150797990800617,0.0148792256101356,
-0.00838015861597521));
#49829=CARTESIAN_POINT('Ctrl Pts',(-0.00149043985841481,0.0148792256101356,
-0.00837479781767868));
#49830=CARTESIAN_POINT('Ctrl Pts',(-0.00105189130935771,0.0148792256101353,
-0.00824076340104341));
#49831=CARTESIAN_POINT('Ctrl Pts',(-0.000592610978165706,0.0148792256101349,
-0.00818111254743533));
#49832=CARTESIAN_POINT('Ctrl Pts',(-0.000133044966495837,0.0148792256101344,
-0.00819713049545326));
#49833=CARTESIAN_POINT('Ctrl Pts',(-9.07585202619122E-5,0.0148792256101343,
-0.00819860436880429));
#49834=CARTESIAN_POINT('Ctrl Pts',(-4.84705149864253E-5,0.0148792256101342,
-0.0082007251339189));
#49835=CARTESIAN_POINT('Ctrl Pts',(-6.19786154605748E-6,0.0148792256101346,
-0.00820349756757392));
#49836=CARTESIAN_POINT('Ctrl Pts',(1.05822949543223E-5,0.0148792256101348,
-0.00820459808686552));
#49837=CARTESIAN_POINT('Ctrl Pts',(2.73591648051649E-5,0.0148792256101349,
-0.00820580129296554));
#49838=CARTESIAN_POINT('Ctrl Pts',(4.41187140605433E-5,0.0148792256101349,
-0.00820710631154845));
#49839=CARTESIAN_POINT('Ctrl Pts',(0.00053266307801239,0.0148792256101353,
-0.00824514787602107));
#49840=CARTESIAN_POINT('Ctrl Pts',(0.00100981843523539,0.0148792256101357,
-0.00836886688399673));
#49841=CARTESIAN_POINT('Ctrl Pts',(0.00144931013511217,0.014879225610136,
-0.00858335194830635));
#49842=CARTESIAN_POINT('Ctrl Pts',(0.00145705942355413,0.014879225610136,
-0.00858713383231075));
#49843=CARTESIAN_POINT('Ctrl Pts',(0.00146479681474301,0.014879225610136,
-0.00859094424863076));
#49844=CARTESIAN_POINT('Ctrl Pts',(0.0014725221409543,0.0148792256101358,
-0.00859478325868824));
#49845=CARTESIAN_POINT('Ctrl Pts',(0.00381143632930178,0.0148792256101254,
-0.0128782269849118));
#49846=CARTESIAN_POINT('Ctrl Pts',(0.00379265690764781,0.0148792256101253,
-0.0130598161005132));
#49847=CARTESIAN_POINT('Ctrl Pts',(0.00376077051328938,0.0148792256101251,
-0.0132393446902149));
#49848=CARTESIAN_POINT('Ctrl Pts',(0.0037154799419432,0.0148792256101249,
-0.0134153953703416));
#49849=CARTESIAN_POINT('Ctrl Pts',(0.00359834182940471,0.0148792256101245,
-0.0138707273250554));
#49850=CARTESIAN_POINT('Ctrl Pts',(0.00339149886618397,0.0148792256101244,
-0.0143027317276141));
#49851=CARTESIAN_POINT('Ctrl Pts',(0.00311742360125872,0.0148792256101242,
-0.014689428358699));
#49852=CARTESIAN_POINT('Ctrl Pts',(0.00310474522725224,0.0148792256101242,
-0.0147073164542091));
#49853=CARTESIAN_POINT('Ctrl Pts',(0.00309192048944817,0.0148792256101242,
-0.0147251109745272));
#49854=CARTESIAN_POINT('Ctrl Pts',(0.00307895095117516,0.0148792256101242,
-0.0147428102674581));
#49855=CARTESIAN_POINT('Ctrl Pts',(0.00306895335665116,0.0148792256101241,
-0.0147564538028223));
#49856=CARTESIAN_POINT('Ctrl Pts',(0.00305887098271552,0.0148792256101241,
-0.0147700389667957));
#49857=CARTESIAN_POINT('Ctrl Pts',(0.00304871004275737,0.0148792256101241,
-0.0147835579687215));
#49858=CARTESIAN_POINT('Ctrl Pts',(0.00275708960701588,0.014879225610124,
-0.0151715552650946));
#49859=CARTESIAN_POINT('Ctrl Pts',(0.00240031763648512,0.0148792256101241,
-0.0155071774786443));
#49860=CARTESIAN_POINT('Ctrl Pts',(0.00199622853595507,0.0148792256101242,
-0.0157734834877795));
#49861=CARTESIAN_POINT('Ctrl Pts',(0.00197766359633304,0.0148792256101242,
-0.01578571830177));
#49862=CARTESIAN_POINT('Ctrl Pts',(0.00195899734363262,0.0148792256101242,
-0.0157978055987294));
#49863=CARTESIAN_POINT('Ctrl Pts',(0.00194023113042077,0.0148792256101242,
-0.0158097433372555));
#49864=CARTESIAN_POINT('Ctrl Pts',(0.00192221297627362,0.0148792256101242,
-0.0158212052134744));
#49865=CARTESIAN_POINT('Ctrl Pts',(0.00190410052124748,0.0148792256101242,
-0.0158325304376092));
#49866=CARTESIAN_POINT('Ctrl Pts',(0.00188591545527795,0.0148792256101242,
-0.0158437048587242));
#49867=CARTESIAN_POINT('Ctrl Pts',(0.00165994072930097,0.0148792256101243,
-0.0159825625760211));
#49868=CARTESIAN_POINT('Ctrl Pts',(0.00142215214426251,0.0148792256101245,
-0.0160986101768173));
#49869=CARTESIAN_POINT('Ctrl Pts',(0.00117533764999415,0.0148792256101246,
-0.0161891562829656));
#49870=CARTESIAN_POINT('Ctrl Pts',(0.000983773707973866,0.0148792256101247,
-0.0162594332295435));
#49871=CARTESIAN_POINT('Ctrl Pts',(0.000786753455184054,0.0148792256101249,
-0.0163143417760653));
#49872=CARTESIAN_POINT('Ctrl Pts',(0.000585895492336925,0.0148792256101251,
-0.016354328533745));
#49873=CARTESIAN_POINT('Ctrl Pts',(0.000547731427410494,0.0148792256101251,
-0.0163619262271332));
#49874=CARTESIAN_POINT('Ctrl Pts',(0.000509428491718366,0.0148792256101251,
-0.0163689842436916));
#49875=CARTESIAN_POINT('Ctrl Pts',(0.000470997421712016,0.0148792256101252,
-0.0163755042835421));
#49876=CARTESIAN_POINT('Ctrl Pts',(0.000452558590985941,0.0148792256101252,
-0.0163786325313664));
#49877=CARTESIAN_POINT('Ctrl Pts',(0.000434090263008574,0.0148792256101252,
-0.0163816369315463));
#49878=CARTESIAN_POINT('Ctrl Pts',(0.000415593619263268,0.0148792256101253,
-0.0163845176364076));
#49879=CARTESIAN_POINT('Ctrl Pts',(0.000272246469694449,0.0148792256101253,
-0.0164068428126023));
#49880=CARTESIAN_POINT('Ctrl Pts',(0.000127921404413201,0.0148792256101256,
-0.0164216327040426));
#49881=CARTESIAN_POINT('Ctrl Pts',(-1.67712264430525E-5,0.0148792256101258,
-0.0164291348700418));
#49882=CARTESIAN_POINT('Ctrl Pts',(-0.000147634627786554,0.0148792256101261,
-0.016435920004532));
#49883=CARTESIAN_POINT('Ctrl Pts',(-0.000278803631839533,0.0148792256101258,
-0.0164367434329844));
#49884=CARTESIAN_POINT('Ctrl Pts',(-0.000409859018321533,0.0148792256101257,
-0.0164317350067629));
#49885=CARTESIAN_POINT('Ctrl Pts',(-0.000631005280122476,0.0148792256101255,
-0.0164232836583208));
#49886=CARTESIAN_POINT('Ctrl Pts',(-0.000851830836900023,0.0148792256101253,
-0.0163982486578753));
#49887=CARTESIAN_POINT('Ctrl Pts',(-0.0010703627002491,0.0148792256101251,
-0.0163569246506869));
#49888=CARTESIAN_POINT('Ctrl Pts',(-0.00111258219104488,0.0148792256101251,
-0.0163489410161066));
#49889=CARTESIAN_POINT('Ctrl Pts',(-0.0011547159952234,0.0148792256101251,
-0.0163403481742521));
#49890=CARTESIAN_POINT('Ctrl Pts',(-0.0011967496481623,0.0148792256101251,
-0.0163311464959581));
#49891=CARTESIAN_POINT('Ctrl Pts',(-0.00175017068631047,0.0148792256101247,
-0.0162099958940444));
#49892=CARTESIAN_POINT('Ctrl Pts',(-0.00227675051008725,0.0148792256101242,
-0.0159865200250432));
#49893=CARTESIAN_POINT('Ctrl Pts',(-0.00274261385400554,0.0148792256101242,
-0.0156656390938508));
#49894=CARTESIAN_POINT('Ctrl Pts',(-0.00275787640298179,0.0148792256101242,
-0.0156551264381723));
#49895=CARTESIAN_POINT('Ctrl Pts',(-0.00277307388134729,0.0148792256101242,
-0.0156445077234186));
#49896=CARTESIAN_POINT('Ctrl Pts',(-0.00278820502685331,0.0148792256101277,
-0.0156337828301188));
#49897=CARTESIAN_POINT('Origin',(0.,0.0148792256101377,-0.0121758532865581));
#49898=CARTESIAN_POINT('Ctrl Pts',(0.00273585250541839,0.0131897093384203,
-0.0149100121428775));
#49899=CARTESIAN_POINT('Ctrl Pts',(0.00185731657271958,0.0132408496933581,
-0.0157891323687994));
#49900=CARTESIAN_POINT('Ctrl Pts',(-0.00079607063101126,0.0133431139771879,
-0.0166247363049608));
#49901=CARTESIAN_POINT('Ctrl Pts',(-0.00411358954646197,0.0134965021899098,
-0.0140558444908958));
#49902=CARTESIAN_POINT('Ctrl Pts',(-0.00388811418891142,0.013649873976586,
-0.00987182162251869));
#49903=CARTESIAN_POINT('Ctrl Pts',(-0.000327275852545556,0.0138032457632622,
-0.00766718327907073));
#49904=CARTESIAN_POINT('Ctrl Pts',(0.0035167017971211,0.0139566175499384,
-0.00933527410552452));
#49905=CARTESIAN_POINT('Ctrl Pts',(0.0043393335020202,0.0141099893366145,
-0.013443238931041));
#49906=CARTESIAN_POINT('Ctrl Pts',(0.00143408777942091,0.0142633611232907,
-0.0164628810402578));
#49907=CARTESIAN_POINT('Ctrl Pts',(-0.00270110084645509,0.0144167329099669,
-0.0157993941062799));
#49908=CARTESIAN_POINT('Ctrl Pts',(-0.00452030709288378,0.0145701046966431,
-0.0120248245767944));
#49909=CARTESIAN_POINT('Ctrl Pts',(-0.00244790251763072,0.0147234846528409,
-0.00837675920613522));
#49910=CARTESIAN_POINT('Ctrl Pts',(0.000322306800181459,0.0148257406801466,
-0.00812604927686857));
#49911=CARTESIAN_POINT('Ctrl Pts',(0.0014715070400914,0.0148768727785604,
-0.00859881810453392));
#49912=CARTESIAN_POINT('Ctrl Pts',(0.00287311792214242,0.0133017513966655,
-0.0150471925844616));
#49913=CARTESIAN_POINT('Ctrl Pts',(0.00195050337019417,0.0133528917516033,
-0.0159704207452677));
#49914=CARTESIAN_POINT('Ctrl Pts',(-0.000836011734082826,0.0134551560354331,
-0.0168479492816357));
#49915=CARTESIAN_POINT('Ctrl Pts',(-0.00431997990639855,0.013608544248155,
-0.0141501689384272));
#49916=CARTESIAN_POINT('Ctrl Pts',(-0.00408319181585019,0.0137619160348312,
-0.00975622187220928));
#49917=CARTESIAN_POINT('Ctrl Pts',(-0.000343696202763411,0.0139152878215074,
-0.00744097062096028));
#49918=CARTESIAN_POINT('Ctrl Pts',(0.00369314461950277,0.0140686596081836,
-0.00919275425686676));
#49919=CARTESIAN_POINT('Ctrl Pts',(0.00455705007127225,0.0142220313948598,
-0.0135068272342465));
#49920=CARTESIAN_POINT('Ctrl Pts',(0.0015060399977043,0.014375403181536,
-0.0166779732829696));
#49921=CARTESIAN_POINT('Ctrl Pts',(-0.00283662267468522,0.0145287749682122,
-0.0159811973429861));
#49922=CARTESIAN_POINT('Ctrl Pts',(-0.00474710361630614,0.0146821467548883,
-0.0120172470415502));
#49923=CARTESIAN_POINT('Ctrl Pts',(-0.0025707206734037,0.0148355267110861,
-0.00818614796847156));
#49924=CARTESIAN_POINT('Ctrl Pts',(0.000338477839063224,0.0149377827383919,
-0.00792285921675396));
#49925=CARTESIAN_POINT('Ctrl Pts',(0.00154533668795086,0.0149889148368055,
-0.00841934818650121));
#49926=CARTESIAN_POINT('Ctrl Pts',(0.00301038333886644,0.0134137934549108,
-0.0151843730260457));
#49927=CARTESIAN_POINT('Ctrl Pts',(0.00204369016766876,0.0134649338098485,
-0.0161517091217361));
#49928=CARTESIAN_POINT('Ctrl Pts',(-0.000875952837154391,0.0135671980936784,
-0.0170711622583103));
#49929=CARTESIAN_POINT('Ctrl Pts',(-0.00452637026633513,0.0137205863064002,
-0.0142444933859585));
#49930=CARTESIAN_POINT('Ctrl Pts',(-0.00427826944278896,0.0138739580930764,
-0.00964062212189988));
#49931=CARTESIAN_POINT('Ctrl Pts',(-0.000360116552981276,0.0140273298797526,
-0.00721475796284981));
#49932=CARTESIAN_POINT('Ctrl Pts',(0.00386958744188443,0.0141807016664288,
-0.00905023440820901));
#49933=CARTESIAN_POINT('Ctrl Pts',(0.00477476664052429,0.014334073453105,
-0.0135704155374519));
#49934=CARTESIAN_POINT('Ctrl Pts',(0.00157799221598771,0.0144874452397812,
-0.0168930655256812));
#49935=CARTESIAN_POINT('Ctrl Pts',(-0.00297214450291535,0.0146408170264574,
-0.0161630005796922));
#49936=CARTESIAN_POINT('Ctrl Pts',(-0.0049739001397285,0.0147941888131336,
-0.0120096695063059));
#49937=CARTESIAN_POINT('Ctrl Pts',(-0.00269353882917668,0.0149475687693314,
-0.0079955367308079));
#49938=CARTESIAN_POINT('Ctrl Pts',(0.000354648877944988,0.0150498247966371,
-0.00771966915663935));
#49939=CARTESIAN_POINT('Ctrl Pts',(0.00161916633581033,0.0151009568950508,
-0.00823987826846848));
#49940=CARTESIAN_POINT('Ctrl Pts',(0.00314764875559048,0.013525835513156,
-0.0153215534676299));
#49941=CARTESIAN_POINT('Ctrl Pts',(0.00213687696514335,0.0135769758680938,
-0.0163329974982044));
#49942=CARTESIAN_POINT('Ctrl Pts',(-0.000915893940225956,0.0136792401519236,
-0.0172943752349851));
#49943=CARTESIAN_POINT('Ctrl Pts',(-0.00473276062627171,0.0138326283646455,
-0.0143388178334899));
#49944=CARTESIAN_POINT('Ctrl Pts',(-0.00447334706972773,0.0139860001513217,
-0.00952502237159047));
#49945=CARTESIAN_POINT('Ctrl Pts',(-0.000376536903199133,0.0141393719379978,
-0.00698854530473934));
#49946=CARTESIAN_POINT('Ctrl Pts',(0.00404603026426609,0.014292743724674,
-0.00890771455955126));
#49947=CARTESIAN_POINT('Ctrl Pts',(0.00499248320977635,0.0144461155113502,
-0.0136340038406574));
#49948=CARTESIAN_POINT('Ctrl Pts',(0.00164994443427111,0.0145994872980264,
-0.017108157768393));
#49949=CARTESIAN_POINT('Ctrl Pts',(-0.00310766633114547,0.0147528590847026,
-0.0163448038163983));
#49950=CARTESIAN_POINT('Ctrl Pts',(-0.00520069666315088,0.0149062308713788,
-0.0120020919710616));
#49951=CARTESIAN_POINT('Ctrl Pts',(-0.00281635698494966,0.0150596108275766,
-0.00780492549314423));
#49952=CARTESIAN_POINT('Ctrl Pts',(0.000370819916826753,0.0151618668548823,
-0.00751647909652474));
#49953=CARTESIAN_POINT('Ctrl Pts',(0.00169299598366981,0.015212998953296,
-0.00806040835043577));
#49954=CARTESIAN_POINT('Ctrl Pts',(-0.00441828210417968,0.0148776665296917,
-0.0126491402494078));
#49955=CARTESIAN_POINT('Ctrl Pts',(-0.00441940407973438,0.0148779235829229,
-0.0126362528549548));
#49956=CARTESIAN_POINT('Ctrl Pts',(-0.004420469123244,0.0148781812985605,
-0.0126233605617627));
#49957=CARTESIAN_POINT('Ctrl Pts',(-0.00442249570517061,0.0148787009257427,
-0.0125974314178203));
#49958=CARTESIAN_POINT('Ctrl Pts',(-0.00442345603009106,0.014878962850937,
-0.0125843945715201));
#49959=CARTESIAN_POINT('Ctrl Pts',(-0.00442435797139694,0.014879225610126,
-0.0125713536543851));
#49960=CARTESIAN_POINT('Ctrl Pts',(-0.00212268276440621,0.0131872148797876,
-0.00826423615450915));
#49961=CARTESIAN_POINT('Ctrl Pts',(-0.000865862298820361,0.0132383524108938,
-0.00758217776404467));
#49962=CARTESIAN_POINT('Ctrl Pts',(0.00233441369372333,0.0133406138708919,
-0.00752903712240916));
#49963=CARTESIAN_POINT('Ctrl Pts',(0.00515297679530513,0.0134939992597821,
-0.011448570453063));
#49964=CARTESIAN_POINT('Ctrl Pts',(0.00353471435351032,0.0136473710464583,
-0.0159900584693641));
#49965=CARTESIAN_POINT('Ctrl Pts',(-0.0011147975591788,0.0138007428331345,
-0.017256387645163));
#49966=CARTESIAN_POINT('Ctrl Pts',(-0.00480898843763011,0.0139541146198107,
-0.0141581177086575));
#49967=CARTESIAN_POINT('Ctrl Pts',(-0.00437176720712775,0.0141074864064868,
-0.00935745063273735));
#49968=CARTESIAN_POINT('Ctrl Pts',(-0.000178648504016178,0.014260858193163,
-0.00697751819934707));
#49969=CARTESIAN_POINT('Ctrl Pts',(0.00416560098168492,0.0144142299798392,
-0.00906295508731642));
#49970=CARTESIAN_POINT('Ctrl Pts',(0.0049368105886653,0.0145676017665154,
-0.013822064507663));
#49971=CARTESIAN_POINT('Ctrl Pts',(0.00145635533370079,0.0147209957524096,
-0.0171681194120463));
#49972=CARTESIAN_POINT('Ctrl Pts',(-0.00168199952693254,0.0148232658094117,
-0.0165374240793895));
#49973=CARTESIAN_POINT('Ctrl Pts',(-0.00279496027439306,0.0148744119375218,
-0.0156391938142977));
#49974=CARTESIAN_POINT('Ctrl Pts',(-0.00203007829900054,0.0132993109570197,
-0.00843488492947408));
#49975=CARTESIAN_POINT('Ctrl Pts',(-0.000828088064892557,0.0133504484881259,
-0.00778258211703734));
#49976=CARTESIAN_POINT('Ctrl Pts',(0.00223257222416043,0.013452709948124,
-0.0077317597967226));
#49977=CARTESIAN_POINT('Ctrl Pts',(0.00492817228406173,0.0136060953370142,
-0.0114802989991858));
#49978=CARTESIAN_POINT('Ctrl Pts',(0.00338050839369504,0.0137594671236905,
-0.0158236594021912));
#49979=CARTESIAN_POINT('Ctrl Pts',(-0.00106616323956478,0.0139128389103666,
-0.0170347435181447));
#49980=CARTESIAN_POINT('Ctrl Pts',(-0.00459919081224947,0.0140662106970428,
-0.0140716391541701));
#49981=CARTESIAN_POINT('Ctrl Pts',(-0.00418104385840945,0.014219582483719,
-0.00948040667470061));
#49982=CARTESIAN_POINT('Ctrl Pts',(-0.000170854758531761,0.0143729542703952,
-0.00720430151799592));
#49983=CARTESIAN_POINT('Ctrl Pts',(0.00398387187054749,0.0145263260570714,
-0.00919875883455404));
#49984=CARTESIAN_POINT('Ctrl Pts',(0.00472143657562934,0.0146796978437475,
-0.0137502466587449));
#49985=CARTESIAN_POINT('Ctrl Pts',(0.00139282016519631,0.0148330918296417,
-0.0169503260877372));
#49986=CARTESIAN_POINT('Ctrl Pts',(-0.00160862037220625,0.0149353618866439,
-0.0163471455609165));
#49987=CARTESIAN_POINT('Ctrl Pts',(-0.00267302693306653,0.014986508014754,
-0.0154881016193325));
#49988=CARTESIAN_POINT('Ctrl Pts',(-0.00193747383359484,0.013411407034252,
-0.00860553370443901));
#49989=CARTESIAN_POINT('Ctrl Pts',(-0.000790313830964761,0.013462544565358,
-0.00798298647003001));
#49990=CARTESIAN_POINT('Ctrl Pts',(0.00213073075459756,0.0135648060253562,
-0.00793448247103606));
#49991=CARTESIAN_POINT('Ctrl Pts',(0.00470336777281834,0.0137181914142464,
-0.0115120275453086));
#49992=CARTESIAN_POINT('Ctrl Pts',(0.00322630243387977,0.0138715632009226,
-0.0156572603350182));
#49993=CARTESIAN_POINT('Ctrl Pts',(-0.00101752891995075,0.0140249349875988,
-0.0168130993911263));
#49994=CARTESIAN_POINT('Ctrl Pts',(-0.00438939318686883,0.014178306774275,
-0.0139851605996826));
#49995=CARTESIAN_POINT('Ctrl Pts',(-0.00399032050969115,0.0143316785609512,
-0.00960336271666387));
#49996=CARTESIAN_POINT('Ctrl Pts',(-0.000163061013047346,0.0144850503476274,
-0.00743108483664477));
#49997=CARTESIAN_POINT('Ctrl Pts',(0.00380214275941005,0.0146384221343036,
-0.00933456258179167));
#49998=CARTESIAN_POINT('Ctrl Pts',(0.00450606256259337,0.0147917939209798,
-0.0136784288098268));
#49999=CARTESIAN_POINT('Ctrl Pts',(0.00132928499669186,0.0149451879068739,
-0.0167325327634281));
#50000=CARTESIAN_POINT('Ctrl Pts',(-0.00153524121747995,0.0150474579638761,
-0.0161568670424437));
#50001=CARTESIAN_POINT('Ctrl Pts',(-0.00255109359174,0.0150986040919861,
-0.0153370094243671));
#50002=CARTESIAN_POINT('Ctrl Pts',(-0.00184486936818917,0.0135235031114842,
-0.00877618247940394));
#50003=CARTESIAN_POINT('Ctrl Pts',(-0.000752539597036957,0.0135746406425903,
-0.00818339082302267));
#50004=CARTESIAN_POINT('Ctrl Pts',(0.00202888928503466,0.0136769021025885,
-0.00813720514534951));
#50005=CARTESIAN_POINT('Ctrl Pts',(0.00447856326157495,0.0138302874914787,
-0.0115437560914314));
#50006=CARTESIAN_POINT('Ctrl Pts',(0.0030720964740645,0.0139836592781549,
-0.0154908612678453));
#50007=CARTESIAN_POINT('Ctrl Pts',(-0.000968894600336737,0.0141370310648311,
-0.0165914552641079));
#50008=CARTESIAN_POINT('Ctrl Pts',(-0.0041795955614882,0.0142904028515072,
-0.0138986820451953));
#50009=CARTESIAN_POINT('Ctrl Pts',(-0.00379959716097288,0.0144437746381834,
-0.00972631875862713));
#50010=CARTESIAN_POINT('Ctrl Pts',(-0.000155267267562925,0.0145971464248596,
-0.00765786815529363));
#50011=CARTESIAN_POINT('Ctrl Pts',(0.0036204136482726,0.0147505182115358,
-0.00947036632902929));
#50012=CARTESIAN_POINT('Ctrl Pts',(0.0042906885495574,0.014903889998212,
-0.0136066109609086));
#50013=CARTESIAN_POINT('Ctrl Pts',(0.00126574982818739,0.0150572839841062,
-0.0165147394391191));
#50014=CARTESIAN_POINT('Ctrl Pts',(-0.00146186206275366,0.0151595540411082,
-0.0159665885239708));
#50015=CARTESIAN_POINT('Ctrl Pts',(-0.00242916025041347,0.0152107001692183,
-0.0151859172294018));
#50016=CARTESIAN_POINT('Origin',(0.,0.0154212256101277,-0.0121758532865581));
#50017=CARTESIAN_POINT('',(-0.0039,0.0154212256101277,-0.0121758532865581));
#50058=UNCERTAINTY_MEASURE_WITH_UNIT(LENGTH_MEASURE(1.E-5),#50082,
'DISTANCE_ACCURACY_VALUE',
'Maximum model space distance between geometric entities at asserted c
onnectivities');
#50059=UNCERTAINTY_MEASURE_WITH_UNIT(LENGTH_MEASURE(1.E-5),#50082,
'DISTANCE_ACCURACY_VALUE',
'Maximum model space distance between geometric entities at asserted c
onnectivities');
#50080=(
GEOMETRIC_REPRESENTATION_CONTEXT(3)
GLOBAL_UNCERTAINTY_ASSIGNED_CONTEXT((#50058))
GLOBAL_UNIT_ASSIGNED_CONTEXT((#50082,#50083,#50084))
REPRESENTATION_CONTEXT('','3D')
);
#50081=(
GEOMETRIC_REPRESENTATION_CONTEXT(3)
GLOBAL_UNCERTAINTY_ASSIGNED_CONTEXT((#50059))
GLOBAL_UNIT_ASSIGNED_CONTEXT((#50082,#50083,#50084))
REPRESENTATION_CONTEXT('','3D')
);
#50082=(
LENGTH_UNIT()
NAMED_UNIT(*)
SI_UNIT($,.METRE.)
);
#50083=(
NAMED_UNIT(*)
PLANE_ANGLE_UNIT()
SI_UNIT($,.RADIAN.)
);
#50084=(
NAMED_UNIT(*)
SI_UNIT($,.STERADIAN.)
SOLID_ANGLE_UNIT()
);
#50105=SHAPE_DEFINITION_REPRESENTATION(#50126,#50167);
#50126=PRODUCT_DEFINITION_SHAPE('',$,#50189);
#50167=SHAPE_REPRESENTATION('',(#10992),#50080);
#50168=PRODUCT_DEFINITION_CONTEXT('part definition',#50233,'design');
#50189=PRODUCT_DEFINITION('Threaded Drive Coupler Insert',
'Threaded Drive Coupler Insert',#50210,#50168);
#50210=PRODUCT_DEFINITION_FORMATION('',$,#50255);
#50233=APPLICATION_CONTEXT('Managed model based 3d engineering');
#50234=PRODUCT_CONTEXT('part definition',#50233,'mechanical');
#50255=PRODUCT('Threaded Drive Coupler Insert',
'Threaded Drive Coupler Insert',
'LEGAL AND USAGE DISCLAIMER: this Data/Model is provided \X2\201C\X0\A
S IS\X2\201D\X0\ for informational and representational only. It is a 
geometric approximation and is NOT engineered, certified, or guarantee
d for dimensional accuracy, exact tolerances, or production-level prec
ision. Vendor disclaims all implied warranties including fitness for a
 particular purpose. DO NOT USE FOR DIRECT PHYSICAL MANUFACTURING, AUT
OMATED PRODUCTION, OR SAFETY-CRITICAL SYSTEMS without independent engi
neering verification and resolution of any design discrepancies.',(#50234));
#50261=PRESENTATION_STYLE_ASSIGNMENT((#50268));
#50268=SURFACE_STYLE_USAGE(.BOTH.,#50275);
#50275=SURFACE_SIDE_STYLE('',(#50282));
#50282=SURFACE_STYLE_FILL_AREA(#50289);
#50289=FILL_AREA_STYLE('Opaque(179,179,179)',(#50296));
#50296=FILL_AREA_STYLE_COLOUR('Opaque(179,179,179)',#50303);
#50303=COLOUR_RGB('Opaque(179,179,179)',0.701960784313725,0.701960784313725,
0.701960784313725);
ENDSEC;
END-ISO-10303-21;
